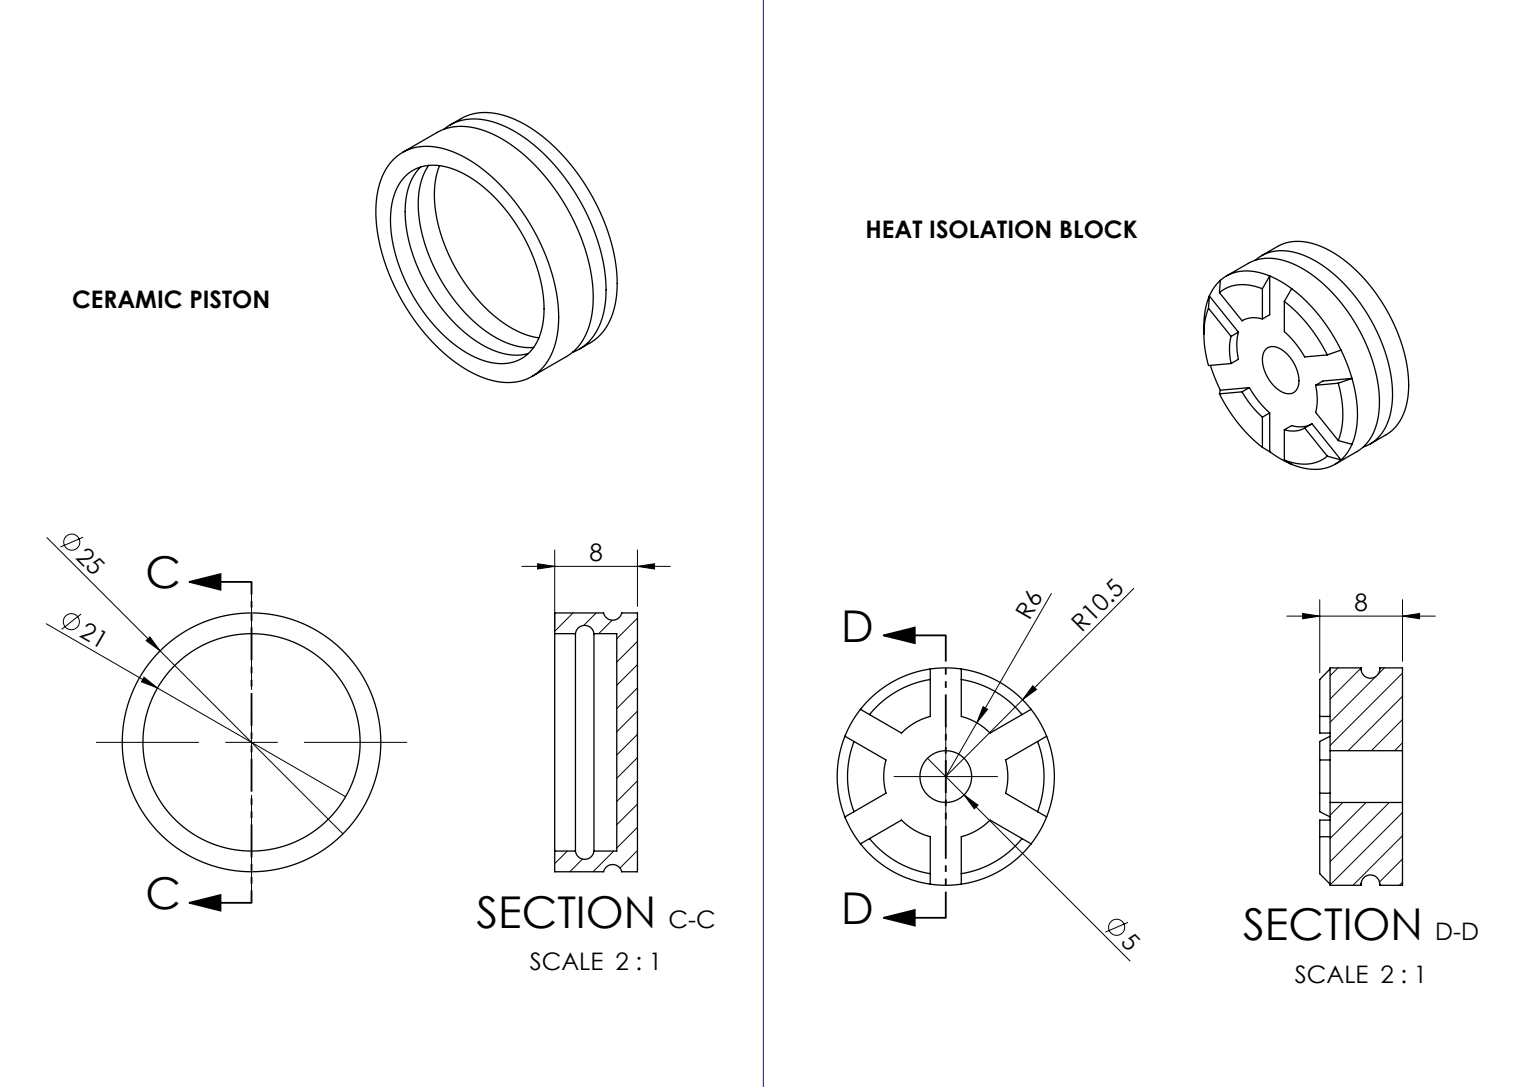
ISO-10303-21;
HEADER;
FILE_DESCRIPTION (('STEP AP214'),
    '1' );
FILE_NAME ('heat isolation block.step',
    '2026-09-24T10:28:59',
    ( '' ),
    ( '' ),
    'SwSTEP 2.0',
    'SolidWorks 2026',
    '' );
FILE_SCHEMA (( 'AUTOMOTIVE_DESIGN' ));
ENDSEC;

DATA;
#9=CARTESIAN_POINT ( 'NONE',  ( -4.281152949374567029, -4.203775615332181914, -2.000000000000000000 ) ) ;
#15=( GEOMETRIC_REPRESENTATION_CONTEXT ( 3 ) GLOBAL_UNCERTAINTY_ASSIGNED_CONTEXT ( ( #3731 ) ) GLOBAL_UNIT_ASSIGNED_CONTEXT ( ( #3713, #4977, #14697 ) ) REPRESENTATION_CONTEXT ( 'NONE', 'WORKASPACE' ) );
#20=CIRCLE ( 'NONE', #5504, 10.50000000000000000 ) ;
#39=CONICAL_SURFACE ( 'NONE', #2378, 9.500000000000001776, 0.7853981633974465026 ) ;
#43=VERTEX_POINT ( 'NONE', #14629 ) ;
#62=CIRCLE ( 'NONE', #4991, 10.50000000000000000 ) ;
#69=DIRECTION ( 'NONE',  ( 0.5000000000000038858, 0.8660254037844363761, 0.000000000000000000 ) ) ;
#71=DIRECTION ( 'NONE',  ( 1.000000000000000000, 0.000000000000000000, 0.000000000000000000 ) ) ;
#73=CARTESIAN_POINT ( 'NONE',  ( 0.000000000000000000, 0.000000000000000000, -2.000000000000000000 ) ) ;
#80=CIRCLE ( 'NONE', #3851, 6.000000000000000888 ) ;
#85=EDGE_LOOP ( 'NONE', ( #16844, #9736, #6237, #10207 ) ) ;
#89=ORIENTED_EDGE ( 'NONE', *, *, #2806, .T. ) ;
#104=CARTESIAN_POINT ( 'NONE',  ( 8.249999999999971578, -6.495190528383328221, -3.000000000000002665 ) ) ;
#107=DIRECTION ( 'NONE',  ( 0.000000000000000000, 0.000000000000000000, -1.000000000000000000 ) ) ;
#128=LINE ( 'NONE', #15357, #5139 ) ;
#130=DIRECTION ( 'NONE',  ( 0.8660254037844432595, 0.4999999999999921174, 0.000000000000000000 ) ) ;
#137=EDGE_CURVE ( 'NONE', #13969, #14024, #12150, .T. ) ;
#143=CARTESIAN_POINT ( 'NONE',  ( 0.000000000000000000, 0.000000000000000000, -3.000000000000000000 ) ) ;
#152=ORIENTED_EDGE ( 'NONE', *, *, #13921, .T. ) ;
#174=ORIENTED_EDGE ( 'NONE', *, *, #13419, .F. ) ;
#189=FACE_OUTER_BOUND ( 'NONE', #16988, .T. ) ;
#198=ORIENTED_EDGE ( 'NONE', *, *, #5351, .T. ) ;
#202=DIRECTION ( 'NONE',  ( -1.000000000000000000, 0.000000000000000000, 0.000000000000000000 ) ) ;
#207=EDGE_LOOP ( 'NONE', ( #11422, #8377, #17595, #13814 ) ) ;
#219=VECTOR ( 'NONE', #12447, 1000.000000000000000 ) ;
#251=CIRCLE ( 'NONE', #10368, 10.50000000000000000 ) ;
#318=ORIENTED_EDGE ( 'NONE', *, *, #17763, .T. ) ;
#357=AXIS2_PLACEMENT_3D ( 'NONE', #9695, #13538, #6726 ) ;
#359=CARTESIAN_POINT ( 'NONE',  ( 0.000000000000000000, 0.000000000000000000, -2.000000000000000000 ) ) ;
#360=AXIS2_PLACEMENT_3D ( 'NONE', #8254, #1099, #13788 ) ;
#369=DIRECTION ( 'NONE',  ( 0.000000000000000000, 0.000000000000000000, 1.000000000000000000 ) ) ;
#371=LINE ( 'NONE', #5878, #16268 ) ;
#388=ADVANCED_FACE ( 'NONE', ( #5520 ), #11038, .F. ) ;
#394=VECTOR ( 'NONE', #8237, 1000.000000000000114 ) ;
#409=CARTESIAN_POINT ( 'NONE',  ( -8.249999999999923617, 6.495190528383386841, -3.000000000000002665 ) ) ;
#415=CARTESIAN_POINT ( 'NONE',  ( -10.50000000000000000, -1.591841644184202181E-21, -6.005572809000082835 ) ) ;
#417=ORIENTED_EDGE ( 'NONE', *, *, #1398, .F. ) ;
#427=CARTESIAN_POINT ( 'NONE',  ( -8.874038404635992805, -3.391377654146690013, -2.000000000000000000 ) ) ;
#439=EDGE_LOOP ( 'NONE', ( #6272, #4236, #9102, #14227 ) ) ;
#467=CARTESIAN_POINT ( 'NONE',  ( -5.781152949374543937, -1.605699403978851247, -2.000000000000000000 ) ) ;
#470=PLANE ( 'NONE',  #13831 ) ;
#480=EDGE_CURVE ( 'NONE', #2781, #625, #723, .T. ) ;
#489=PLANE ( 'NONE',  #1672 ) ;
#504=DIRECTION ( 'NONE',  ( 1.000000000000000000, 0.000000000000000000, 0.000000000000000000 ) ) ;
#509=ORIENTED_EDGE ( 'NONE', *, *, #6536, .T. ) ;
#515=CARTESIAN_POINT ( 'NONE',  ( 1.500000000000000000, -10.39230484541326405, -3.000000000000000000 ) ) ;
#544=CARTESIAN_POINT ( 'NONE',  ( 0.000000000000000000, 0.000000000000000000, -10.00000000000000000 ) ) ;
#557=EDGE_CURVE ( 'NONE', #11479, #14024, #4933, .T. ) ;
#571=DIRECTION ( 'NONE',  ( 1.000000000000000000, 0.000000000000000000, -0.000000000000000000 ) ) ;
#578=EDGE_CURVE ( 'NONE', #729, #4780, #14420, .T. ) ;
#579=VERTEX_POINT ( 'NONE', #6435 ) ;
#601=CARTESIAN_POINT ( 'NONE',  ( 1.296864337298335788E-21, -1.182044466681725685E-21, -6.899999999999998579 ) ) ;
#606=DIRECTION ( 'NONE',  ( 0.4999999999999921174, -0.8660254037844432595, -0.000000000000000000 ) ) ;
#625=VERTEX_POINT ( 'NONE', #4973 ) ;
#634=CARTESIAN_POINT ( 'NONE',  ( 5.781152949374520844, -1.605699403978932294, -1.901951201008075243 ) ) ;
#643=ORIENTED_EDGE ( 'NONE', *, *, #10821, .T. ) ;
#667=VECTOR ( 'NONE', #5113, 1000.000000000000000 ) ;
#674=LINE ( 'NONE', #6104, #12815 ) ;
#676=DIRECTION ( 'NONE',  ( 1.000000000000000000, 0.000000000000000000, -0.000000000000000000 ) ) ;
#688=DIRECTION ( 'NONE',  ( 0.000000000000000000, 0.000000000000000000, 1.000000000000000000 ) ) ;
#700=CARTESIAN_POINT ( 'NONE',  ( 2.500000000000000000, 0.000000000000000000, -10.00000000000000000 ) ) ;
#710=EDGE_CURVE ( 'NONE', #12766, #3366, #5509, .T. ) ;
#723=LINE ( 'NONE', #1918, #13063 ) ;
#729=VERTEX_POINT ( 'NONE', #6905 ) ;
#744=FACE_OUTER_BOUND ( 'NONE', #10937, .T. ) ;
#749=LINE ( 'NONE', #17278, #4040 ) ;
#752=EDGE_CURVE ( 'NONE', #1869, #2438, #6375, .T. ) ;
#764=CARTESIAN_POINT ( 'NONE',  ( -4.281152949374478212, 4.203775615332272508, -3.000000000000000888 ) ) ;
#819=CARTESIAN_POINT ( 'NONE',  ( -7.958171371210956302, 6.326703190994831694, -2.666481567098320404 ) ) ;
#821=EDGE_LOOP ( 'NONE', ( #12913, #198, #11384, #8365 ) ) ;
#842=AXIS2_PLACEMENT_3D ( 'NONE', #9935, #3246, #7424 ) ;
#848=CIRCLE ( 'NONE', #14764, 9.500000000000001776 ) ;
#849=FACE_OUTER_BOUND ( 'NONE', #85, .T. ) ;
#851=CARTESIAN_POINT ( 'NONE',  ( 0.000000000000000000, 0.000000000000000000, -3.000000000000002665 ) ) ;
#912=ORIENTED_EDGE ( 'NONE', *, *, #15355, .F. ) ;
#915=ADVANCED_FACE ( 'NONE', ( #1453 ), #39, .T. ) ;
#932=FACE_OUTER_BOUND ( 'NONE', #17119, .T. ) ;
#937=CIRCLE ( 'NONE', #357, 6.000000000000000888 ) ;
#940=VECTOR ( 'NONE', #5062, 1000.000000000000000 ) ;
#946=CARTESIAN_POINT ( 'NONE',  ( 1.500000000000000000, -11.00000000000000000, -9.708203932499369415 ) ) ;
#1001=DIRECTION ( 'NONE',  ( 0.000000000000000000, 0.000000000000000000, -1.000000000000000000 ) ) ;
#1049=ORIENTED_EDGE ( 'NONE', *, *, #11408, .F. ) ;
#1060=CARTESIAN_POINT ( 'NONE',  ( -10.50000000000000000, 0.000000000000000000, -2.000000000000000000 ) ) ;
#1069=VERTEX_POINT ( 'NONE', #8885 ) ;
#1099=DIRECTION ( 'NONE',  ( -0.000000000000000000, -0.000000000000000000, 1.000000000000000000 ) ) ;
#1136=AXIS2_PLACEMENT_3D ( 'NONE', #7243, #8688, #3068 ) ;
#1187=EDGE_LOOP ( 'NONE', ( #16383, #1379, #6856, #3698 ) ) ;
#1190=LINE ( 'NONE', #7567, #15018 ) ;
#1192=AXIS2_PLACEMENT_3D ( 'NONE', #16349, #13436, #5076 ) ;
#1198=VERTEX_POINT ( 'NONE', #8051 ) ;
#1209=AXIS2_PLACEMENT_3D ( 'NONE', #2238, #17500, #17400 ) ;
#1235=CIRCLE ( 'NONE', #11336, 2.500000000000000000 ) ;
#1240=ADVANCED_FACE ( 'NONE', ( #2709 ), #17880, .T. ) ;
#1258=DIRECTION ( 'NONE',  ( -0.8660254037844397068, -0.4999999999999981126, 0.000000000000000000 ) ) ;
#1288=EDGE_LOOP ( 'NONE', ( #15134, #15555, #15815, #8257 ) ) ;
#1290=CARTESIAN_POINT ( 'NONE',  ( -1.500000000000000000, -10.39230484541326405, -3.000000000000002665 ) ) ;
#1307=DIRECTION ( 'NONE',  ( 0.8660254037844397068, 0.4999999999999981126, -0.000000000000000000 ) ) ;
#1308=CARTESIAN_POINT ( 'NONE',  ( 0.000000000000000000, 0.000000000000000000, -2.000000000000000000 ) ) ;
#1332=ORIENTED_EDGE ( 'NONE', *, *, #12922, .F. ) ;
#1344=FACE_OUTER_BOUND ( 'NONE', #5620, .T. ) ;
#1350=ORIENTED_EDGE ( 'NONE', *, *, #12982, .T. ) ;
#1360=CARTESIAN_POINT ( 'NONE',  ( 9.750000000000010658, 3.897114317029950037, -3.000000000000002665 ) ) ;
#1368=AXIS2_PLACEMENT_3D ( 'NONE', #5699, #11216, #16788 ) ;
#1372=CARTESIAN_POINT ( 'NONE',  ( 7.958171371211001599, -6.326703190994774850, -2.666481567098319960 ) ) ;
#1379=ORIENTED_EDGE ( 'NONE', *, *, #5330, .F. ) ;
#1392=DIRECTION ( 'NONE',  ( 1.000000000000000000, 0.000000000000000000, 0.000000000000000000 ) ) ;
#1398=EDGE_CURVE ( 'NONE', #9792, #11171, #4666, .T. ) ;
#1408=PRODUCT_DEFINITION_CONTEXT ( 'detailed design', #12580, 'design' ) ;
#1414=CARTESIAN_POINT ( 'NONE',  ( 10.37836969302994028, -0.6704047395399680420, -6.899999999999998579 ) ) ;
#1421=VERTEX_POINT ( 'NONE', #13936 ) ;
#1431=AXIS2_PLACEMENT_3D ( 'NONE', #10215, #17040, #3248 ) ;
#1453=FACE_OUTER_BOUND ( 'NONE', #15787, .T. ) ;
#1455=CARTESIAN_POINT ( 'NONE',  ( -1.500000000000000000, 10.39230484541326227, -3.000000000000000000 ) ) ;
#1470=AXIS2_PLACEMENT_3D ( 'NONE', #15599, #1647, #12691 ) ;
#1472=CARTESIAN_POINT ( 'NONE',  ( -1.499999999999999778, 9.380831519646861238, -2.000000000000000000 ) ) ;
#1512=EDGE_CURVE ( 'NONE', #11483, #15072, #14540, .T. ) ;
#1523=CARTESIAN_POINT ( 'NONE',  ( 1.499999999999999778, -9.718191103688257115, -2.333127728361105380 ) ) ;
#1526=ORIENTED_EDGE ( 'NONE', *, *, #7540, .T. ) ;
#1553=DIRECTION ( 'NONE',  ( 0.000000000000000000, 0.000000000000000000, -1.000000000000000000 ) ) ;
#1566=ORIENTED_EDGE ( 'NONE', *, *, #10647, .T. ) ;
#1572=VERTEX_POINT ( 'NONE', #5185 ) ;
#1580=CARTESIAN_POINT ( 'NONE',  ( 5.781152949374531502, 1.605699403978890771, -1.901951201008075243 ) ) ;
#1600=ADVANCED_FACE ( 'NONE', ( #9886 ), #12895, .F. ) ;
#1615=VERTEX_POINT ( 'NONE', #8632 ) ;
#1626=DIRECTION ( 'NONE',  ( 0.000000000000000000, 0.000000000000000000, -1.000000000000000000 ) ) ;
#1647=DIRECTION ( 'NONE',  ( 0.4999999999999921174, -0.8660254037844432595, -0.000000000000000000 ) ) ;
#1655=CARTESIAN_POINT ( 'NONE',  ( -1.500000000000000000, 10.05532945112458698, -2.666480854966546854 ) ) ;
#1668=ADVANCED_FACE ( 'NONE', ( #744 ), #12214, .F. ) ;
#1672=AXIS2_PLACEMENT_3D ( 'NONE', #7393, #12994, #6000 ) ;
#1699=CARTESIAN_POINT ( 'NONE',  ( 1.499999999999999778, -9.380831519646861238, -2.000000000000000000 ) ) ;
#1700=EDGE_CURVE ( 'NONE', #17480, #7830, #17463, .T. ) ;
#1727=FACE_OUTER_BOUND ( 'NONE', #3816, .T. ) ;
#1738=CARTESIAN_POINT ( 'NONE',  ( -8.776279441628744848, 6.799038105676760146, -11.72793873352925331 ) ) ;
#1745=CARTESIAN_POINT ( 'NONE',  ( 1.500000000000000666, 5.809475019311125976, -3.000000000000000000 ) ) ;
#1757=PLANE ( 'NONE',  #3505 ) ;
#1768=CARTESIAN_POINT ( 'NONE',  ( 0.000000000000000000, 0.000000000000000000, -2.000000000000000000 ) ) ;
#1772=DIRECTION ( 'NONE',  ( 1.224646799147353207E-16, -1.000000000000000000, 0.000000000000000000 ) ) ;
#1786=DIRECTION ( 'NONE',  ( -0.8660254037844397068, -0.4999999999999981126, 0.000000000000000000 ) ) ;
#1798=CARTESIAN_POINT ( 'NONE',  ( -10.37836969302994028, 0.6704047395399693743, -6.899999999999998579 ) ) ;
#1802=AXIS2_PLACEMENT_3D ( 'NONE', #10064, #17179, #202 ) ;
#1809=PLANE ( 'NONE',  #1136 ) ;
#1842=VECTOR ( 'NONE', #5538, 1000.000000000000000 ) ;
#1843=AXIS2_PLACEMENT_3D ( 'NONE', #12222, #9657, #2789 ) ;
#1849=CIRCLE ( 'NONE', #1431, 10.50000000000000000 ) ;
#1851=EDGE_LOOP ( 'NONE', ( #4202, #12524, #6400, #11426 ) ) ;
#1862=CIRCLE ( 'NONE', #6762, 9.500000000000000000 ) ;
#1867=ORIENTED_EDGE ( 'NONE', *, *, #13233, .T. ) ;
#1869=VERTEX_POINT ( 'NONE', #1455 ) ;
#1875=CIRCLE ( 'NONE', #3312, 2.500000000000000000 ) ;
#1918=CARTESIAN_POINT ( 'NONE',  ( 8.776279441628840772, 6.799038105676637578, -3.000000000000000888 ) ) ;
#1929=DIRECTION ( 'NONE',  ( -0.000000000000000000, -0.000000000000000000, -1.000000000000000000 ) ) ;
#1936=ADVANCED_FACE ( 'NONE', ( #10861 ), #2733, .F. ) ;
#1938=ORIENTED_EDGE ( 'NONE', *, *, #9820, .F. ) ;
#1984=CARTESIAN_POINT ( 'NONE',  ( 0.000000000000000000, 0.000000000000000000, -2.000000000000000000 ) ) ;
#1993=ORIENTED_EDGE ( 'NONE', *, *, #14425, .F. ) ;
#1996=EDGE_CURVE ( 'NONE', #14070, #1615, #10473, .T. ) ;
#2030=DIRECTION ( 'NONE',  ( -1.000000000000000000, 0.000000000000000000, 0.000000000000000000 ) ) ;
#2038=CYLINDRICAL_SURFACE ( 'NONE', #14415, 10.50000000000000000 ) ;
#2040=DIRECTION ( 'NONE',  ( 1.000000000000000000, 0.000000000000000000, 0.000000000000000000 ) ) ;
#2042=DIRECTION ( 'NONE',  ( 0.000000000000000000, 0.000000000000000000, -1.000000000000000000 ) ) ;
#2053=DIRECTION ( 'NONE',  ( 1.000000000000000000, 0.000000000000000000, 0.000000000000000000 ) ) ;
#2071=LINE ( 'NONE', #700, #12556 ) ;
#2076=ADVANCED_FACE ( 'NONE', ( #5791 ), #16001, .T. ) ;
#2083=DIRECTION ( 'NONE',  ( -1.000000000000000000, 0.000000000000000000, 0.000000000000000000 ) ) ;
#2099=CIRCLE ( 'NONE', #13645, 10.50000000000000000 ) ;
#2109=EDGE_CURVE ( 'NONE', #3845, #13908, #12877, .T. ) ;
#2116=EDGE_LOOP ( 'NONE', ( #14184, #10060, #9084, #13984 ) ) ;
#2125=CIRCLE ( 'NONE', #4141, 10.50000000000000000 ) ;
#2129=VECTOR ( 'NONE', #4034, 999.9999999999998863 ) ;
#2141=CARTESIAN_POINT ( 'NONE',  ( 0.000000000000000000, 0.000000000000000000, -3.000000000000002665 ) ) ;
#2172=CYLINDRICAL_SURFACE ( 'NONE', #7782, 6.000000000000000888 ) ;
#2184=DIRECTION ( 'NONE',  ( -0.000000000000000000, -0.000000000000000000, -1.000000000000000000 ) ) ;
#2196=EDGE_LOOP ( 'NONE', ( #15610, #7635, #5937, #16842 ) ) ;
#2220=EDGE_CURVE ( 'NONE', #15040, #7588, #15871, .T. ) ;
#2226=VERTEX_POINT ( 'NONE', #13147 ) ;
#2231=EDGE_CURVE ( 'NONE', #15452, #4832, #62, .T. ) ;
#2238=CARTESIAN_POINT ( 'NONE',  ( 8.472608240843633681E-22, -7.722472891792491889E-22, -7.794427190999915211 ) ) ;
#2248=CARTESIAN_POINT ( 'NONE',  ( 0.000000000000000000, 0.000000000000000000, -3.000000000000002665 ) ) ;
#2250=CARTESIAN_POINT ( 'NONE',  ( 10.27627944162880702, -4.200961894323389956, -11.72793873352923910 ) ) ;
#2280=FILL_AREA_STYLE ('',( #9238 ) ) ;
#2308=ADVANCED_FACE ( 'NONE', ( #1344 ), #13506, .T. ) ;
#2309=CIRCLE ( 'NONE', #4601, 10.50000000000000000 ) ;
#2319=DIRECTION ( 'NONE',  ( 1.000000000000000000, 4.440892098500626951E-15, 0.000000000000000000 ) ) ;
#2322=AXIS2_PLACEMENT_3D ( 'NONE', #6054, #3437, #5876 ) ;
#2343=DIRECTION ( 'NONE',  ( 0.5000000000000038858, 0.8660254037844363761, 0.000000000000000000 ) ) ;
#2346=DIRECTION ( 'NONE',  ( -1.000000000000000000, 0.000000000000000000, 0.000000000000000000 ) ) ;
#2371=CARTESIAN_POINT ( 'NONE',  ( 0.000000000000000000, 0.000000000000000000, -3.000000000000002665 ) ) ;
#2374=SURFACE_STYLE_USAGE ( .BOTH. , #14785 ) ;
#2378=AXIS2_PLACEMENT_3D ( 'NONE', #12332, #17897, #10945 ) ;
#2389=AXIS2_PLACEMENT_3D ( 'NONE', #16083, #3561, #10523 ) ;
#2421=ORIENTED_EDGE ( 'NONE', *, *, #3769, .F. ) ;
#2438=VERTEX_POINT ( 'NONE', #16490 ) ;
#2454=( NAMED_UNIT ( * ) PLANE_ANGLE_UNIT ( ) SI_UNIT ( $, .RADIAN. ) );
#2462=EDGE_CURVE ( 'NONE', #14411, #17313, #11338, .T. ) ;
#2529=LINE ( 'NONE', #15127, #394 ) ;
#2540=ORIENTED_EDGE ( 'NONE', *, *, #5351, .F. ) ;
#2546=CARTESIAN_POINT ( 'NONE',  ( 8.776279441628796363, -6.799038105676699750, -3.000000000000000888 ) ) ;
#2558=DIRECTION ( 'NONE',  ( 1.000000000000000000, 7.105427357601001859E-15, 0.000000000000000000 ) ) ;
#2566=AXIS2_PLACEMENT_3D ( 'NONE', #17401, #3402, #11731 ) ;
#2637=CARTESIAN_POINT ( 'NONE',  ( 8.874038404635971489, 3.391377654146752629, -2.000000000000000000 ) ) ;
#2645=EDGE_CURVE ( 'NONE', #9826, #1069, #3570, .T. ) ;
#2653=AXIS2_PLACEMENT_3D ( 'NONE', #11618, #6546, #17738 ) ;
#2669=AXIS2_PLACEMENT_3D ( 'NONE', #11406, #1553, #12604 ) ;
#2709=FACE_OUTER_BOUND ( 'NONE', #4089, .T. ) ;
#2715=SHAPE_REPRESENTATION_RELATIONSHIP ( 'NONE' , 'NONE' ,  #12598, #7018 ) ;
#2733=CYLINDRICAL_SURFACE ( 'NONE', #360, 2.500000000000000000 ) ;
#2740=CARTESIAN_POINT ( 'NONE',  ( 4.281152949374537720, 4.203775615332211224, -3.000000000000000888 ) ) ;
#2780=ORIENTED_EDGE ( 'NONE', *, *, #13626, .F. ) ;
#2781=VERTEX_POINT ( 'NONE', #2740 ) ;
#2789=DIRECTION ( 'NONE',  ( -0.9979201627913402151, 0.06446199418653550395, 5.311609029246448998E-22 ) ) ;
#2798=CARTESIAN_POINT ( 'NONE',  ( -1.500000000000000222, -9.718191103688257115, -2.333127728361105824 ) ) ;
#2806=EDGE_CURVE ( 'NONE', #13908, #625, #6456, .T. ) ;
#2839=VERTEX_POINT ( 'NONE', #3278 ) ;
#2852=VECTOR ( 'NONE', #15204, 1000.000000000000000 ) ;
#2868=CARTESIAN_POINT ( 'NONE',  ( 8.776279441628840772, 6.799038105676637578, -11.72793873352922489 ) ) ;
#2873=DIRECTION ( 'NONE',  ( -0.8660254037844363761, 0.5000000000000038858, 0.000000000000000000 ) ) ;
#2910=ORIENTED_EDGE ( 'NONE', *, *, #10359, .T. ) ;
#2921=CARTESIAN_POINT ( 'NONE',  ( -9.480241546517731877, 0.6123889447720874957, -6.899999999999998579 ) ) ;
#2957=AXIS2_PLACEMENT_3D ( 'NONE', #1798, #10206, #9832 ) ;
#2969=ORIENTED_EDGE ( 'NONE', *, *, #10235, .T. ) ;
#2987=DIRECTION ( 'NONE',  ( 1.000000000000000000, 0.000000000000000000, 0.000000000000000000 ) ) ;
#2988=ADVANCED_FACE ( 'NONE', ( #8616 ), #14148, .T. ) ;
#3008=CARTESIAN_POINT ( 'NONE',  ( 7.666200962222293747, -6.158133996769738161, -2.333128398347827481 ) ) ;
#3062=DIRECTION ( 'NONE',  ( -0.000000000000000000, -0.000000000000000000, -1.000000000000000000 ) ) ;
#3068=DIRECTION ( 'NONE',  ( -0.8660254037844397068, -0.4999999999999981126, 0.000000000000000000 ) ) ;
#3101=DIRECTION ( 'NONE',  ( 0.000000000000000000, 0.000000000000000000, 1.000000000000000000 ) ) ;
#3104=AXIS2_PLACEMENT_3D ( 'NONE', #11983, #16358, #17566 ) ;
#3160=ORIENTED_EDGE ( 'NONE', *, *, #10235, .F. ) ;
#3205=AXIS2_PLACEMENT_3D ( 'NONE', #10231, #10312, #10043 ) ;
#3220=SHAPE_DEFINITION_REPRESENTATION ( #17387, #12598 ) ;
#3229=VECTOR ( 'NONE', #17641, 999.9999999999998863 ) ;
#3246=DIRECTION ( 'NONE',  ( 0.000000000000000000, 0.000000000000000000, -1.000000000000000000 ) ) ;
#3248=DIRECTION ( 'NONE',  ( 1.000000000000000000, 0.000000000000000000, 0.000000000000000000 ) ) ;
#3278=CARTESIAN_POINT ( 'NONE',  ( -4.281152949374479100, 4.203775615332271620, -2.000000000000000000 ) ) ;
#3292=EDGE_CURVE ( 'NONE', #11171, #14411, #8219, .T. ) ;
#3306=DIRECTION ( 'NONE',  ( 0.000000000000000000, 0.000000000000000000, -1.000000000000000000 ) ) ;
#3309=DIRECTION ( 'NONE',  ( -0.000000000000000000, -0.000000000000000000, -1.000000000000000000 ) ) ;
#3312=AXIS2_PLACEMENT_3D ( 'NONE', #5444, #12434, #16617 ) ;
#3319=CARTESIAN_POINT ( 'NONE',  ( -7.958171371211089529, -6.326703190994665604, -2.666481567098319516 ) ) ;
#3331=DIRECTION ( 'NONE',  ( -0.000000000000000000, -0.000000000000000000, 1.000000000000000000 ) ) ;
#3344=ORIENTED_EDGE ( 'NONE', *, *, #5310, .T. ) ;
#3357=EDGE_CURVE ( 'NONE', #1615, #14070, #251, .T. ) ;
#3362=FACE_OUTER_BOUND ( 'NONE', #5487, .T. ) ;
#3366=VERTEX_POINT ( 'NONE', #427 ) ;
#3367=ADVANCED_FACE ( 'NONE', ( #11823 ), #11513, .F. ) ;
#3388=CARTESIAN_POINT ( 'NONE',  ( 10.50000000000000000, 1.285879139104720831E-15, -2.000000000000000000 ) ) ;
#3395=LINE ( 'NONE', #7572, #1842 ) ;
#3402=DIRECTION ( 'NONE',  ( -5.026720092345836698E-22, 4.581671729415424240E-22, -1.000000000000000000 ) ) ;
#3404=VECTOR ( 'NONE', #7432, 1000.000000000000000 ) ;
#3405=ORIENTED_EDGE ( 'NONE', *, *, #10870, .F. ) ;
#3422=FACE_OUTER_BOUND ( 'NONE', #8222, .T. ) ;
#3437=DIRECTION ( 'NONE',  ( 0.000000000000000000, 0.000000000000000000, -1.000000000000000000 ) ) ;
#3471=CARTESIAN_POINT ( 'NONE',  ( -2.500000000000000000, 3.061616997868383141E-16, -10.00000000000000000 ) ) ;
#3505=AXIS2_PLACEMENT_3D ( 'NONE', #14357, #12986, #571 ) ;
#3506=DIRECTION ( 'NONE',  ( 1.000000000000000000, 0.000000000000000000, 0.000000000000000000 ) ) ;
#3525=ORIENTED_EDGE ( 'NONE', *, *, #17843, .F. ) ;
#3540=AXIS2_PLACEMENT_3D ( 'NONE', #544, #16784, #14056 ) ;
#3554=AXIS2_PLACEMENT_3D ( 'NONE', #6267, #14796, #11882 ) ;
#3561=DIRECTION ( 'NONE',  ( -5.026720092345836698E-22, 4.581671729415424240E-22, -1.000000000000000000 ) ) ;
#3570=LINE ( 'NONE', #3471, #8184 ) ;
#3575=AXIS2_PLACEMENT_3D ( 'NONE', #5095, #17575, #9272 ) ;
#3577=ORIENTED_EDGE ( 'NONE', *, *, #11050, .T. ) ;
#3589=DIRECTION ( 'NONE',  ( 1.000000000000000000, 0.000000000000000000, 0.000000000000000000 ) ) ;
#3600=DIRECTION ( 'NONE',  ( -1.000000000000000000, 0.000000000000000000, 0.000000000000000000 ) ) ;
#3609=PLANE ( 'NONE',  #13979 ) ;
#3615=PRODUCT ( 'heat isolation block', 'heat isolation block', '', ( #13914 ) ) ;
#3643=EDGE_LOOP ( 'NONE', ( #3916, #14619, #4515, #16461, #2780 ) ) ;
#3665=CARTESIAN_POINT ( 'NONE',  ( -9.458171371211065548, -3.728626979641334493, -2.666481567098320404 ) ) ;
#3684=CARTESIAN_POINT ( 'NONE',  ( 1.500000000000000000, 10.05532945112459053, -2.666480854966549519 ) ) ;
#3697=ORIENTED_EDGE ( 'NONE', *, *, #578, .F. ) ;
#3698=ORIENTED_EDGE ( 'NONE', *, *, #14726, .F. ) ;
#3713=( LENGTH_UNIT ( ) NAMED_UNIT ( * ) SI_UNIT ( .MILLI., .METRE. ) );
#3715=CIRCLE ( 'NONE', #6012, 0.9000000000000003553 ) ;
#3731=UNCERTAINTY_MEASURE_WITH_UNIT (LENGTH_MEASURE( 1.000000000000000082E-05 ), #3713, 'distance_accuracy_value', 'NONE');
#3752=CARTESIAN_POINT ( 'NONE',  ( -1.500000000000000000, -11.00000000000000000, -2.000000000000000000 ) ) ;
#3758=CARTESIAN_POINT ( 'NONE',  ( 7.374038404635976818, 5.989453865500072638, -2.000000000000000000 ) ) ;
#3759=B_SPLINE_CURVE_WITH_KNOTS ( 'NONE', 3,
 ( #17890, #13856, #2798, #10934 ),
 .UNSPECIFIED., .F., .F.,
 ( 4, 4 ),
 ( 0.007932485430080135971, 0.009354825709699443950 ),
 .UNSPECIFIED. ) ;
#3769=EDGE_CURVE ( 'NONE', #15072, #12450, #6094, .T. ) ;
#3773=VERTEX_POINT ( 'NONE', #5910 ) ;
#3775=CARTESIAN_POINT ( 'NONE',  ( 1.500000000000000000, 10.39230484541326227, -3.000000000000000000 ) ) ;
#3785=CARTESIAN_POINT ( 'NONE',  ( 10.50000000000000000, 1.285879139104720831E-15, -3.000000000000002665 ) ) ;
#3802=ADVANCED_FACE ( 'NONE', ( #15624 ), #14272, .T. ) ;
#3811=VECTOR ( 'NONE', #15051, 999.9999999999998863 ) ;
#3816=EDGE_LOOP ( 'NONE', ( #4598, #10832, #4008, #10200 ) ) ;
#3819=ORIENTED_EDGE ( 'NONE', *, *, #4860, .T. ) ;
#3830=AXIS2_PLACEMENT_3D ( 'NONE', #6269, #7906, #11885 ) ;
#3845=VERTEX_POINT ( 'NONE', #1745 ) ;
#3848=VECTOR ( 'NONE', #1772, 1000.000000000000000 ) ;
#3851=AXIS2_PLACEMENT_3D ( 'NONE', #17013, #7216, #8477 ) ;
#3857=AXIS2_PLACEMENT_3D ( 'NONE', #11830, #606, #13117 ) ;
#3887=DIRECTION ( 'NONE',  ( 0.000000000000000000, 0.000000000000000000, 1.000000000000000000 ) ) ;
#3916=ORIENTED_EDGE ( 'NONE', *, *, #4860, .F. ) ;
#3957=CARTESIAN_POINT ( 'NONE',  ( 1.500000000000000222, 9.380831519646861238, -2.000000000000000000 ) ) ;
#3964=ORIENTED_EDGE ( 'NONE', *, *, #16776, .T. ) ;
#3971=VECTOR ( 'NONE', #16088, 1000.000000000000000 ) ;
#3986=CIRCLE ( 'NONE', #10905, 10.50000000000000000 ) ;
#4008=ORIENTED_EDGE ( 'NONE', *, *, #12945, .F. ) ;
#4017=ORIENTED_EDGE ( 'NONE', *, *, #15259, .F. ) ;
#4020=CARTESIAN_POINT ( 'NONE',  ( -10.50000000000000000, 0.000000000000000000, -10.00000000000000000 ) ) ;
#4034=DIRECTION ( 'NONE',  ( -0.7071067811865462405, 0.000000000000000000, -0.7071067811865489050 ) ) ;
#4040=VECTOR ( 'NONE', #15896, 1000.000000000000114 ) ;
#4047=AXIS2_PLACEMENT_3D ( 'NONE', #5466, #15185, #6927 ) ;
#4048=ORIENTED_EDGE ( 'NONE', *, *, #15785, .T. ) ;
#4056=DIRECTION ( 'NONE',  ( 1.000000000000000000, 0.000000000000000000, 0.000000000000000000 ) ) ;
#4069=EDGE_CURVE ( 'NONE', #15072, #2226, #11486, .T. ) ;
#4078=LINE ( 'NONE', #2546, #3229 ) ;
#4089=EDGE_LOOP ( 'NONE', ( #7110, #11157, #11633, #17145, #10471, #8655 ) ) ;
#4099=EDGE_CURVE ( 'NONE', #1198, #579, #8316, .T. ) ;
#4107=EDGE_CURVE ( 'NONE', #1572, #17008, #13634, .T. ) ;
#4131=CARTESIAN_POINT ( 'NONE',  ( 0.000000000000000000, 0.000000000000000000, -1.901951201008075243 ) ) ;
#4141=AXIS2_PLACEMENT_3D ( 'NONE', #2141, #2042, #11634 ) ;
#4147=EDGE_CURVE ( 'NONE', #11147, #14109, #3986, .T. ) ;
#4191=EDGE_CURVE ( 'NONE', #14530, #1198, #7387, .T. ) ;
#4202=ORIENTED_EDGE ( 'NONE', *, *, #7943, .T. ) ;
#4236=ORIENTED_EDGE ( 'NONE', *, *, #15879, .T. ) ;
#4252=FACE_OUTER_BOUND ( 'NONE', #12699, .T. ) ;
#4255=ORIENTED_EDGE ( 'NONE', *, *, #9354, .F. ) ;
#4295=VECTOR ( 'NONE', #9727, 1000.000000000000000 ) ;
#4335=CIRCLE ( 'NONE', #8972, 6.000000000000000888 ) ;
#4379=CIRCLE ( 'NONE', #16830, 10.50000000000000000 ) ;
#4433=EDGE_LOOP ( 'NONE', ( #12591, #16245 ) ) ;
#4468=ORIENTED_EDGE ( 'NONE', *, *, #10158, .T. ) ;
#4484=EDGE_CURVE ( 'NONE', #13130, #1572, #5053, .T. ) ;
#4499=FACE_OUTER_BOUND ( 'NONE', #12923, .T. ) ;
#4515=ORIENTED_EDGE ( 'NONE', *, *, #1512, .F. ) ;
#4534=CARTESIAN_POINT ( 'NONE',  ( 0.000000000000000000, 0.000000000000000000, -2.000000000000000000 ) ) ;
#4544=ORIENTED_EDGE ( 'NONE', *, *, #13626, .T. ) ;
#4555=CONICAL_SURFACE ( 'NONE', #1368, 9.500000000000001776, 0.7853981633974465026 ) ;
#4557=CARTESIAN_POINT ( 'NONE',  ( 8.472608240843633681E-22, -7.722472891792491889E-22, -7.794427190999915211 ) ) ;
#4593=VERTEX_POINT ( 'NONE', #9713 ) ;
#4598=ORIENTED_EDGE ( 'NONE', *, *, #6536, .F. ) ;
#4601=AXIS2_PLACEMENT_3D ( 'NONE', #2371, #13507, #7889 ) ;
#4625=LINE ( 'NONE', #16793, #6902 ) ;
#4639=EDGE_CURVE ( 'NONE', #9144, #579, #128, .T. ) ;
#4654=ORIENTED_EDGE ( 'NONE', *, *, #752, .T. ) ;
#4655=CARTESIAN_POINT ( 'NONE',  ( 1.500000000000000000, -11.00000000000000000, -3.000000000000000000 ) ) ;
#4657=CARTESIAN_POINT ( 'NONE',  ( 0.000000000000000000, 0.000000000000000000, -1.901951201008075243 ) ) ;
#4666=CIRCLE ( 'NONE', #14810, 6.000000000000000888 ) ;
#4701=DIRECTION ( 'NONE',  ( -1.000000000000000000, 0.000000000000000000, 0.000000000000000000 ) ) ;
#4734=ADVANCED_FACE ( 'NONE', ( #14367 ), #489, .T. ) ;
#4735=DIRECTION ( 'NONE',  ( -0.000000000000000000, -0.000000000000000000, -1.000000000000000000 ) ) ;
#4738=ADVANCED_FACE ( 'NONE', ( #17098 ), #2038, .T. ) ;
#4739=ORIENTED_EDGE ( 'NONE', *, *, #15462, .F. ) ;
#4749=CARTESIAN_POINT ( 'NONE',  ( 0.000000000000000000, 0.000000000000000000, -2.000000000000000000 ) ) ;
#4750=CARTESIAN_POINT ( 'NONE',  ( -6.000000000000000888, 0.000000000000000000, -3.000000000000000000 ) ) ;
#4765=CARTESIAN_POINT ( 'NONE',  ( 1.500000000000000222, 9.380831519646861238, -2.000000000000000000 ) ) ;
#4780=VERTEX_POINT ( 'NONE', #10177 ) ;
#4788=EDGE_CURVE ( 'NONE', #12819, #43, #8619, .T. ) ;
#4814=CARTESIAN_POINT ( 'NONE',  ( -4.281152949374566141, -4.203775615332181026, -3.000000000000000888 ) ) ;
#4827=FACE_OUTER_BOUND ( 'NONE', #4433, .T. ) ;
#4832=VERTEX_POINT ( 'NONE', #409 ) ;
#4859=LINE ( 'NONE', #1060, #11852 ) ;
#4860=EDGE_CURVE ( 'NONE', #2226, #8959, #8646, .T. ) ;
#4883=FACE_OUTER_BOUND ( 'NONE', #8544, .T. ) ;
#4904=B_SPLINE_CURVE_WITH_KNOTS ( 'NONE', 3,
 ( #11646, #3319, #8932, #14474 ),
 .UNSPECIFIED., .F., .F.,
 ( 4, 4 ),
 ( 2.843119637691541009E-07, 0.001422633878257847061 ),
 .UNSPECIFIED. ) ;
#4915=ORIENTED_EDGE ( 'NONE', *, *, #5443, .F. ) ;
#4918=CARTESIAN_POINT ( 'NONE',  ( 0.000000000000000000, 0.000000000000000000, -2.000000000000000000 ) ) ;
#4933=CIRCLE ( 'NONE', #3205, 6.000000000000000888 ) ;
#4946=DIRECTION ( 'NONE',  ( -1.000000000000000000, 0.000000000000000000, 0.000000000000000000 ) ) ;
#4955=CARTESIAN_POINT ( 'NONE',  ( -7.374038404636016786, -5.989453865500021124, -2.000000000000000000 ) ) ;
#4961=ORIENTED_EDGE ( 'NONE', *, *, #3357, .T. ) ;
#4973=CARTESIAN_POINT ( 'NONE',  ( 8.250000000000014211, 6.495190528383269601, -3.000000000000000000 ) ) ;
#4977=( NAMED_UNIT ( * ) PLANE_ANGLE_UNIT ( ) SI_UNIT ( $, .RADIAN. ) );
#4980=VECTOR ( 'NONE', #6063, 1000.000000000000000 ) ;
#4991=AXIS2_PLACEMENT_3D ( 'NONE', #10582, #1001, #14613 ) ;
#5053=LINE ( 'NONE', #11676, #3404 ) ;
#5062=DIRECTION ( 'NONE',  ( 1.224646799147353207E-16, -1.000000000000000000, 0.000000000000000000 ) ) ;
#5076=DIRECTION ( 'NONE',  ( -1.000000000000000000, 0.000000000000000000, 0.000000000000000000 ) ) ;
#5092=CARTESIAN_POINT ( 'NONE',  ( 9.166200962222307069, -3.560057785416429255, -2.333128398347826593 ) ) ;
#5095=CARTESIAN_POINT ( 'NONE',  ( 0.000000000000000000, 0.000000000000000000, 0.000000000000000000 ) ) ;
#5096=DIRECTION ( 'NONE',  ( -1.224646799147353207E-16, 1.000000000000000000, 0.000000000000000000 ) ) ;
#5099=EDGE_CURVE ( 'NONE', #5285, #7960, #17353, .T. ) ;
#5104=ORIENTED_EDGE ( 'NONE', *, *, #12475, .T. ) ;
#5113=DIRECTION ( 'NONE',  ( 0.000000000000000000, 0.000000000000000000, -1.000000000000000000 ) ) ;
#5123=CARTESIAN_POINT ( 'NONE',  ( -5.781152949374542160, -1.605699403978850803, -3.000000000000000888 ) ) ;
#5134=ORIENTED_EDGE ( 'NONE', *, *, #16914, .T. ) ;
#5139=VECTOR ( 'NONE', #5641, 1000.000000000000000 ) ;
#5145=CARTESIAN_POINT ( 'NONE',  ( 0.000000000000000000, 0.000000000000000000, -2.000000000000000000 ) ) ;
#5155=DIRECTION ( 'NONE',  ( 1.000000000000000000, -1.776356839400250780E-14, 0.000000000000000000 ) ) ;
#5185=CARTESIAN_POINT ( 'NONE',  ( 5.781152949374531502, 1.605699403978890993, -2.000000000000000000 ) ) ;
#5195=ORIENTED_EDGE ( 'NONE', *, *, #12475, .F. ) ;
#5219=EDGE_LOOP ( 'NONE', ( #8639, #7984, #174, #17028 ) ) ;
#5247=VECTOR ( 'NONE', #14814, 1000.000000000000000 ) ;
#5285=VERTEX_POINT ( 'NONE', #17435 ) ;
#5293=CARTESIAN_POINT ( 'NONE',  ( 0.000000000000000000, 0.000000000000000000, -2.000000000000000000 ) ) ;
#5310=EDGE_CURVE ( 'NONE', #1421, #7830, #14508, .T. ) ;
#5312=CARTESIAN_POINT ( 'NONE',  ( 0.000000000000000000, 0.000000000000000000, -2.000000000000000000 ) ) ;
#5329=ORIENTED_EDGE ( 'NONE', *, *, #13805, .T. ) ;
#5330=EDGE_CURVE ( 'NONE', #1198, #10066, #8966, .T. ) ;
#5333=CARTESIAN_POINT ( 'NONE',  ( 9.458171371211037126, 3.728626979641400219, -2.666481567098320848 ) ) ;
#5344=SURFACE_STYLE_USAGE ( .BOTH. , #12609 ) ;
#5351=EDGE_CURVE ( 'NONE', #9800, #15040, #17670, .T. ) ;
#5379=ORIENTED_EDGE ( 'NONE', *, *, #7811, .F. ) ;
#5433=VERTEX_POINT ( 'NONE', #9401 ) ;
#5437=PRESENTATION_STYLE_ASSIGNMENT (( #5344 ) ) ;
#5438=CARTESIAN_POINT ( 'NONE',  ( 7.374038404635931521, -5.989453865500120600, -2.000000000000000000 ) ) ;
#5443=EDGE_CURVE ( 'NONE', #8628, #11479, #10917, .T. ) ;
#5444=CARTESIAN_POINT ( 'NONE',  ( 0.000000000000000000, 0.000000000000000000, -10.00000000000000000 ) ) ;
#5466=CARTESIAN_POINT ( 'NONE',  ( 0.000000000000000000, 0.000000000000000000, -3.000000000000002665 ) ) ;
#5468=CARTESIAN_POINT ( 'NONE',  ( -10.27627944162877505, 4.200961894323461010, -11.72793873352925331 ) ) ;
#5481=AXIS2_PLACEMENT_3D ( 'NONE', #4657, #12637, #9993 ) ;
#5487=EDGE_LOOP ( 'NONE', ( #4654, #17307, #14687, #14006 ) ) ;
#5497=CARTESIAN_POINT ( 'NONE',  ( -4.281152949374479100, 4.203775615332273397, -1.901951201008075243 ) ) ;
#5504=AXIS2_PLACEMENT_3D ( 'NONE', #16220, #9049, #11845 ) ;
#5508=ADVANCED_FACE ( 'NONE', ( #7235 ), #12576, .T. ) ;
#5509=CIRCLE ( 'NONE', #15663, 9.500000000000001776 ) ;
#5520=FACE_OUTER_BOUND ( 'NONE', #7894, .T. ) ;
#5538=DIRECTION ( 'NONE',  ( 1.224646799147353207E-16, -1.000000000000000000, 0.000000000000000000 ) ) ;
#5543=AXIS2_PLACEMENT_3D ( 'NONE', #1414, #10999, #9646 ) ;
#5566=LINE ( 'NONE', #11084, #16772 ) ;
#5585=DIRECTION ( 'NONE',  ( 1.000000000000000000, 8.881784197001252323E-16, 0.000000000000000000 ) ) ;
#5613=DIRECTION ( 'NONE',  ( 1.000000000000000000, 0.000000000000000000, -0.000000000000000000 ) ) ;
#5620=EDGE_LOOP ( 'NONE', ( #7306, #4544, #7105, #16938 ) ) ;
#5641=DIRECTION ( 'NONE',  ( -1.224646799147353207E-16, 1.000000000000000000, 0.000000000000000000 ) ) ;
#5654=CYLINDRICAL_SURFACE ( 'NONE', #12999, 6.000000000000000888 ) ;
#5681=CARTESIAN_POINT ( 'NONE',  ( 0.000000000000000000, 0.000000000000000000, -2.000000000000000000 ) ) ;
#5690=PLANE ( 'NONE',  #10166 ) ;
#5699=CARTESIAN_POINT ( 'NONE',  ( 0.000000000000000000, 0.000000000000000000, -2.000000000000000000 ) ) ;
#5727=ADVANCED_FACE ( 'NONE', ( #14596 ), #2172, .F. ) ;
#5733=ORIENTED_EDGE ( 'NONE', *, *, #17759, .F. ) ;
#5750=ORIENTED_EDGE ( 'NONE', *, *, #11050, .F. ) ;
#5791=FACE_OUTER_BOUND ( 'NONE', #439, .T. ) ;
#5817=ORIENTED_EDGE ( 'NONE', *, *, #16914, .F. ) ;
#5823=VECTOR ( 'NONE', #1786, 1000.000000000000000 ) ;
#5856=CARTESIAN_POINT ( 'NONE',  ( -8.776279441628885181, -6.799038105676576293, -3.000000000000000888 ) ) ;
#5862=FACE_OUTER_BOUND ( 'NONE', #16136, .T. ) ;
#5876=DIRECTION ( 'NONE',  ( 1.000000000000000000, 0.000000000000000000, 0.000000000000000000 ) ) ;
#5878=CARTESIAN_POINT ( 'NONE',  ( -5.781152949374542160, -1.605699403978851247, -1.901951201008075243 ) ) ;
#5887=CARTESIAN_POINT ( 'NONE',  ( 10.27627944162880702, -4.200961894323389956, -2.000000000000000000 ) ) ;
#5900=ORIENTED_EDGE ( 'NONE', *, *, #4484, .F. ) ;
#5910=CARTESIAN_POINT ( 'NONE',  ( -8.874038404635921751, 3.391377654146875642, -2.000000000000000000 ) ) ;
#5919=EDGE_LOOP ( 'NONE', ( #9185, #7628, #13149, #4915 ) ) ;
#5922=ORIENTED_EDGE ( 'NONE', *, *, #16179, .T. ) ;
#5937=ORIENTED_EDGE ( 'NONE', *, *, #17446, .T. ) ;
#5975=DIRECTION ( 'NONE',  ( -0.5000000000000099920, -0.8660254037844329345, 0.000000000000000000 ) ) ;
#6000=DIRECTION ( 'NONE',  ( 1.000000000000000000, 0.000000000000000000, -0.000000000000000000 ) ) ;
#6006=DIRECTION ( 'NONE',  ( 0.000000000000000000, 0.000000000000000000, -1.000000000000000000 ) ) ;
#6012=AXIS2_PLACEMENT_3D ( 'NONE', #15788, #11600, #6260 ) ;
#6035=LINE ( 'NONE', #7421, #14552 ) ;
#6046=AXIS2_PLACEMENT_3D ( 'NONE', #4918, #8070, #2040 ) ;
#6054=CARTESIAN_POINT ( 'NONE',  ( 0.000000000000000000, 0.000000000000000000, -3.000000000000002665 ) ) ;
#6055=DIRECTION ( 'NONE',  ( -5.026720092345836698E-22, 4.581671729415424240E-22, -1.000000000000000000 ) ) ;
#6063=DIRECTION ( 'NONE',  ( -1.224646799147353207E-16, 1.000000000000000000, 0.000000000000000000 ) ) ;
#6072=EDGE_CURVE ( 'NONE', #4832, #1869, #2309, .T. ) ;
#6088=ORIENTED_EDGE ( 'NONE', *, *, #17358, .T. ) ;
#6094=LINE ( 'NONE', #14551, #10038 ) ;
#6104=CARTESIAN_POINT ( 'NONE',  ( 1.500000000000000666, 5.809475019311125976, -1.901951201008075243 ) ) ;
#6106=CARTESIAN_POINT ( 'NONE',  ( -9.749999999999953815, 3.897114317030088149, -3.000000000000000000 ) ) ;
#6150=ORIENTED_EDGE ( 'NONE', *, *, #8192, .T. ) ;
#6153=CIRCLE ( 'NONE', #2957, 0.9000000000000003553 ) ;
#6159=EDGE_CURVE ( 'NONE', #2839, #7960, #12398, .T. ) ;
#6170=DIRECTION ( 'NONE',  ( 1.000000000000000000, 0.000000000000000000, 0.000000000000000000 ) ) ;
#6172=ADVANCED_FACE ( 'NONE', ( #5862 ), #14217, .F. ) ;
#6205=ADVANCED_FACE ( 'NONE', ( #10214 ), #1809, .T. ) ;
#6223=ORIENTED_EDGE ( 'NONE', *, *, #6159, .F. ) ;
#6237=ORIENTED_EDGE ( 'NONE', *, *, #14569, .T. ) ;
#6260=DIRECTION ( 'NONE',  ( 0.9979201627913403261, -0.06446199418653547619, 0.000000000000000000 ) ) ;
#6267=CARTESIAN_POINT ( 'NONE',  ( 0.000000000000000000, 0.000000000000000000, -3.000000000000000000 ) ) ;
#6268=ORIENTED_EDGE ( 'NONE', *, *, #15189, .T. ) ;
#6269=CARTESIAN_POINT ( 'NONE',  ( 1.746467850512308208E-21, -1.591841644184202181E-21, -6.005572809000082835 ) ) ;
#6272=ORIENTED_EDGE ( 'NONE', *, *, #710, .F. ) ;
#6349=CARTESIAN_POINT ( 'NONE',  ( -7.374038404635891553, 5.989453865500174778, -2.000000000000000000 ) ) ;
#6375=B_SPLINE_CURVE_WITH_KNOTS ( 'NONE', 3,
 ( #15245, #1655, #9610, #1472 ),
 .UNSPECIFIED., .F., .F.,
 ( 4, 4 ),
 ( 0.007932485430080135971, 0.009354825709699440481 ),
 .UNSPECIFIED. ) ;
#6380=PLANE ( 'NONE',  #11317 ) ;
#6388=AXIS2_PLACEMENT_3D ( 'NONE', #13116, #10632, #11655 ) ;
#6390=FACE_OUTER_BOUND ( 'NONE', #11076, .T. ) ;
#6392=B_SPLINE_CURVE_WITH_KNOTS ( 'NONE', 3,
 ( #3775, #3684, #9299, #4765 ),
 .UNSPECIFIED., .F., .F.,
 ( 4, 4 ),
 ( 0.007932485430080137706, 0.009354825709699442216 ),
 .UNSPECIFIED. ) ;
#6397=AXIS2_PLACEMENT_3D ( 'NONE', #14054, #12684, #9681 ) ;
#6398=ORIENTED_EDGE ( 'NONE', *, *, #11670, .F. ) ;
#6400=ORIENTED_EDGE ( 'NONE', *, *, #5443, .T. ) ;
#6419=FACE_OUTER_BOUND ( 'NONE', #3643, .T. ) ;
#6420=STYLED_ITEM ( 'NONE', ( #5437 ), #11123 ) ;
#6425=EDGE_CURVE ( 'NONE', #3366, #10034, #7395, .T. ) ;
#6435=CARTESIAN_POINT ( 'NONE',  ( 1.499999999999999334, -5.809475019311126864, -2.000000000000000000 ) ) ;
#6441=CIRCLE ( 'NONE', #10757, 2.500000000000000000 ) ;
#6455=ORIENTED_EDGE ( 'NONE', *, *, #15879, .F. ) ;
#6456=CIRCLE ( 'NONE', #14271, 10.50000000000000000 ) ;
#6462=ORIENTED_EDGE ( 'NONE', *, *, #2462, .T. ) ;
#6468=FACE_BOUND ( 'NONE', #12862, .T. ) ;
#6482=CARTESIAN_POINT ( 'NONE',  ( -9.166200962222356807, -3.560057785416302689, -2.333128398347827481 ) ) ;
#6536=EDGE_CURVE ( 'NONE', #17313, #11147, #1190, .T. ) ;
#6546=DIRECTION ( 'NONE',  ( -0.000000000000000000, -0.000000000000000000, -1.000000000000000000 ) ) ;
#6554=ORIENTED_EDGE ( 'NONE', *, *, #15595, .F. ) ;
#6572=CARTESIAN_POINT ( 'NONE',  ( 1.500000000000000000, -10.39230484541326405, -3.000000000000000000 ) ) ;
#6575=ORIENTED_EDGE ( 'NONE', *, *, #6849, .T. ) ;
#6618=EDGE_CURVE ( 'NONE', #10285, #17504, #13870, .T. ) ;
#6653=AXIS2_PLACEMENT_3D ( 'NONE', #4749, #8927, #3589 ) ;
#6664=VERTEX_POINT ( 'NONE', #10266 ) ;
#6667=VECTOR ( 'NONE', #15281, 1000.000000000000114 ) ;
#6677=VERTEX_POINT ( 'NONE', #7739 ) ;
#6689=FACE_OUTER_BOUND ( 'NONE', #10611, .T. ) ;
#6716=AXIS2_PLACEMENT_3D ( 'NONE', #11636, #10356, #676 ) ;
#6720=EDGE_CURVE ( 'NONE', #11483, #13130, #17211, .T. ) ;
#6722=CIRCLE ( 'NONE', #12243, 0.9000000000000003553 ) ;
#6726=DIRECTION ( 'NONE',  ( 1.000000000000000000, 0.000000000000000000, 0.000000000000000000 ) ) ;
#6728=ORIENTED_EDGE ( 'NONE', *, *, #8192, .F. ) ;
#6734=AXIS2_PLACEMENT_3D ( 'NONE', #5293, #12460, #15269 ) ;
#6736=CIRCLE ( 'NONE', #1209, 10.50000000000000000 ) ;
#6745=CIRCLE ( 'NONE', #13428, 10.50000000000000000 ) ;
#6760=DIRECTION ( 'NONE',  ( -1.000000000000000000, 0.000000000000000000, 0.000000000000000000 ) ) ;
#6762=AXIS2_PLACEMENT_3D ( 'NONE', #601, #17911, #3600 ) ;
#6771=ORIENTED_EDGE ( 'NONE', *, *, #9109, .T. ) ;
#6777=ORIENTED_EDGE ( 'NONE', *, *, #4107, .F. ) ;
#6802=EDGE_CURVE ( 'NONE', #1572, #729, #4335, .T. ) ;
#6839=CARTESIAN_POINT ( 'NONE',  ( 1.500000000000000666, 5.809475019311125976, -2.000000000000000000 ) ) ;
#6842=DIRECTION ( 'NONE',  ( 0.8660254037844329345, -0.5000000000000099920, 0.000000000000000000 ) ) ;
#6849=EDGE_CURVE ( 'NONE', #14109, #6677, #13309, .T. ) ;
#6856=ORIENTED_EDGE ( 'NONE', *, *, #4191, .F. ) ;
#6857=B_SPLINE_CURVE_WITH_KNOTS ( 'NONE', 3,
 ( #6106, #9106, #9014, #10270 ),
 .UNSPECIFIED., .F., .F.,
 ( 4, 4 ),
 ( 2.843119637709864978E-07, 0.001422633878257846410 ),
 .UNSPECIFIED. ) ;
#6863=DIRECTION ( 'NONE',  ( 0.000000000000000000, 0.000000000000000000, 1.000000000000000000 ) ) ;
#6896=FILL_AREA_STYLE ('',( #13791 ) ) ;
#6902=VECTOR ( 'NONE', #107, 1000.000000000000000 ) ;
#6903=VERTEX_POINT ( 'NONE', #8881 ) ;
#6905=CARTESIAN_POINT ( 'NONE',  ( 5.781152949374518180, -1.605699403978931405, -2.000000000000000000 ) ) ;
#6919=EDGE_LOOP ( 'NONE', ( #11825, #17770, #643, #16034, #16052, #6771, #15361, #15224, #9583, #89, #10076 ) ) ;
#6927=DIRECTION ( 'NONE',  ( 1.000000000000000000, 3.552713678800500929E-15, 0.000000000000000000 ) ) ;
#6959=( GEOMETRIC_REPRESENTATION_CONTEXT ( 3 ) GLOBAL_UNCERTAINTY_ASSIGNED_CONTEXT ( ( #8610 ) ) GLOBAL_UNIT_ASSIGNED_CONTEXT ( ( #13425, #2454, #9749 ) ) REPRESENTATION_CONTEXT ( 'NONE', 'WORKASPACE' ) );
#6973=ORIENTED_EDGE ( 'NONE', *, *, #7540, .F. ) ;
#6976=EDGE_CURVE ( 'NONE', #14024, #9359, #11552, .T. ) ;
#7014=CARTESIAN_POINT ( 'NONE',  ( 0.000000000000000000, 0.000000000000000000, -3.000000000000002665 ) ) ;
#7015=CIRCLE ( 'NONE', #5543, 0.9000000000000003553 ) ;
#7018=ADVANCED_BREP_SHAPE_REPRESENTATION ( '', ( #11123, #3575 ), #15 ) ;
#7034=CARTESIAN_POINT ( 'NONE',  ( 8.250000000000014211, 6.495190528383269601, -3.000000000000000000 ) ) ;
#7037=CARTESIAN_POINT ( 'NONE',  ( -9.500000000000001776, 0.000000000000000000, -2.000000000000000000 ) ) ;
#7041=CONICAL_SURFACE ( 'NONE', #16319, 9.500000000000001776, 0.7853981633974465026 ) ;
#7103=B_SPLINE_CURVE_WITH_KNOTS ( 'NONE', 3,
 ( #7034, #11249, #11535, #10184 ),
 .UNSPECIFIED., .F., .F.,
 ( 4, 4 ),
 ( 2.843119637714455897E-07, 0.001422633878257845976 ),
 .UNSPECIFIED. ) ;
#7105=ORIENTED_EDGE ( 'NONE', *, *, #4484, .T. ) ;
#7110=ORIENTED_EDGE ( 'NONE', *, *, #8996, .F. ) ;
#7113=DIRECTION ( 'NONE',  ( 1.000000000000000000, 0.000000000000000000, 0.000000000000000000 ) ) ;
#7161=DIRECTION ( 'NONE',  ( -1.000000000000000000, 0.000000000000000000, 0.000000000000000000 ) ) ;
#7181=CARTESIAN_POINT ( 'NONE',  ( 4.281152949374508410, -4.203775615332241422, -3.000000000000000888 ) ) ;
#7185=AXIS2_PLACEMENT_3D ( 'NONE', #1308, #10884, #9705 ) ;
#7207=AXIS2_PLACEMENT_3D ( 'NONE', #12658, #69, #2873 ) ;
#7208=AXIS2_PLACEMENT_3D ( 'NONE', #1738, #5975, #11499 ) ;
#7213=ORIENTED_EDGE ( 'NONE', *, *, #7589, .T. ) ;
#7216=DIRECTION ( 'NONE',  ( 0.000000000000000000, 0.000000000000000000, 1.000000000000000000 ) ) ;
#7228=AXIS2_PLACEMENT_3D ( 'NONE', #12033, #3887, #16230 ) ;
#7235=FACE_OUTER_BOUND ( 'NONE', #1187, .T. ) ;
#7243=CARTESIAN_POINT ( 'NONE',  ( 10.27627944162883544, 4.200961894323318013, -11.72793873352922489 ) ) ;
#7266=AXIS2_PLACEMENT_3D ( 'NONE', #7604, #17609, #2083 ) ;
#7268=CARTESIAN_POINT ( 'NONE',  ( -1.500000000000000000, 11.00000000000000000, -9.708203932499369415 ) ) ;
#7283=AXIS2_PLACEMENT_3D ( 'NONE', #13763, #6863, #12394 ) ;
#7306=ORIENTED_EDGE ( 'NONE', *, *, #10158, .F. ) ;
#7366=LINE ( 'NONE', #5887, #13345 ) ;
#7386=CARTESIAN_POINT ( 'NONE',  ( -10.50000000000000000, 0.000000000000000000, -7.794427190999915211 ) ) ;
#7387=LINE ( 'NONE', #9981, #11186 ) ;
#7389=CARTESIAN_POINT ( 'NONE',  ( 0.000000000000000000, 0.000000000000000000, -2.000000000000000000 ) ) ;
#7392=EDGE_CURVE ( 'NONE', #2839, #13145, #9825, .T. ) ;
#7393=CARTESIAN_POINT ( 'NONE',  ( 0.000000000000000000, 0.000000000000000000, -2.000000000000000000 ) ) ;
#7395=LINE ( 'NONE', #12818, #17379 ) ;
#7399=FACE_OUTER_BOUND ( 'NONE', #15267, .T. ) ;
#7402=ORIENTED_EDGE ( 'NONE', *, *, #8369, .F. ) ;
#7407=CARTESIAN_POINT ( 'NONE',  ( 4.281152949374537720, 4.203775615332211224, -2.000000000000000000 ) ) ;
#7409=DIRECTION ( 'NONE',  ( -0.000000000000000000, -0.000000000000000000, -1.000000000000000000 ) ) ;
#7421=CARTESIAN_POINT ( 'NONE',  ( -8.776279441628744848, 6.799038105676760146, -3.000000000000000888 ) ) ;
#7424=DIRECTION ( 'NONE',  ( -1.000000000000000000, 0.000000000000000000, 0.000000000000000000 ) ) ;
#7432=DIRECTION ( 'NONE',  ( -0.8660254037844397068, -0.4999999999999981126, 0.000000000000000000 ) ) ;
#7436=CARTESIAN_POINT ( 'NONE',  ( 10.50000000000000000, 1.285879139104720831E-15, -6.005572809000082835 ) ) ;
#7459=AXIS2_PLACEMENT_3D ( 'NONE', #7389, #12903, #12159 ) ;
#7463=DIRECTION ( 'NONE',  ( 5.026720092345836698E-22, -4.581671729415424240E-22, 1.000000000000000000 ) ) ;
#7471=DIRECTION ( 'NONE',  ( -5.026720092345836698E-22, 4.581671729415424240E-22, -1.000000000000000000 ) ) ;
#7484=CARTESIAN_POINT ( 'NONE',  ( -6.000000000000000888, 0.000000000000000000, -2.000000000000000000 ) ) ;
#7503=DIRECTION ( 'NONE',  ( -0.8660254037844329345, 0.5000000000000099920, 0.000000000000000000 ) ) ;
#7518=ORIENTED_EDGE ( 'NONE', *, *, #14055, .F. ) ;
#7534=ORIENTED_EDGE ( 'NONE', *, *, #16958, .T. ) ;
#7540=EDGE_CURVE ( 'NONE', #13908, #15040, #6392, .T. ) ;
#7566=LINE ( 'NONE', #3388, #12746 ) ;
#7567=CARTESIAN_POINT ( 'NONE',  ( -1.500000000000000000, -11.00000000000000000, -3.000000000000000000 ) ) ;
#7568=ORIENTED_EDGE ( 'NONE', *, *, #4788, .F. ) ;
#7572=CARTESIAN_POINT ( 'NONE',  ( -1.500000000000000000, 11.00000000000000000, -2.000000000000000000 ) ) ;
#7588=VERTEX_POINT ( 'NONE', #6839 ) ;
#7589=EDGE_CURVE ( 'NONE', #6677, #1421, #11863, .T. ) ;
#7598=CARTESIAN_POINT ( 'NONE',  ( -5.781152949374509298, 1.605699403978973372, -2.000000000000000000 ) ) ;
#7604=CARTESIAN_POINT ( 'NONE',  ( 0.000000000000000000, 0.000000000000000000, -2.000000000000000000 ) ) ;
#7616=CARTESIAN_POINT ( 'NONE',  ( 4.281152949374507521, -4.203775615332241422, -1.901951201008075243 ) ) ;
#7626=SURFACE_STYLE_FILL_AREA ( #2280 ) ;
#7628=ORIENTED_EDGE ( 'NONE', *, *, #137, .T. ) ;
#7635=ORIENTED_EDGE ( 'NONE', *, *, #16853, .F. ) ;
#7645=ORIENTED_EDGE ( 'NONE', *, *, #15322, .T. ) ;
#7686=DIRECTION ( 'NONE',  ( 0.000000000000000000, 0.000000000000000000, -1.000000000000000000 ) ) ;
#7739=CARTESIAN_POINT ( 'NONE',  ( -9.750000000000035527, -3.897114317029883868, -3.000000000000002665 ) ) ;
#7782=AXIS2_PLACEMENT_3D ( 'NONE', #10296, #7686, #2346 ) ;
#7806=AXIS2_PLACEMENT_3D ( 'NONE', #5681, #12671, #7161 ) ;
#7811=EDGE_CURVE ( 'NONE', #13145, #5285, #10084, .T. ) ;
#7814=ADVANCED_FACE ( 'NONE', ( #7399 ), #14285, .F. ) ;
#7830=VERTEX_POINT ( 'NONE', #415 ) ;
#7834=EDGE_CURVE ( 'NONE', #625, #9800, #7103, .T. ) ;
#7835=DIRECTION ( 'NONE',  ( 0.000000000000000000, 0.000000000000000000, -1.000000000000000000 ) ) ;
#7861=DIRECTION ( 'NONE',  ( -0.8660254037844363761, 0.5000000000000038858, 0.000000000000000000 ) ) ;
#7889=DIRECTION ( 'NONE',  ( 1.000000000000000000, 1.776356839400250465E-15, 0.000000000000000000 ) ) ;
#7894=EDGE_LOOP ( 'NONE', ( #10062, #14436, #17532, #1049 ) ) ;
#7897=CARTESIAN_POINT ( 'NONE',  ( -7.666200962222251114, 6.158133996769793228, -2.333128398347828369 ) ) ;
#7906=DIRECTION ( 'NONE',  ( 5.026720092345836698E-22, -4.581671729415424240E-22, 1.000000000000000000 ) ) ;
#7909=DIRECTION ( 'NONE',  ( 1.000000000000000000, 0.000000000000000000, 0.000000000000000000 ) ) ;
#7943=EDGE_CURVE ( 'NONE', #15452, #3773, #6857, .T. ) ;
#7959=ADVANCED_FACE ( 'NONE', ( #13186, #4827 ), #14565, .F. ) ;
#7960=VERTEX_POINT ( 'NONE', #764 ) ;
#7984=ORIENTED_EDGE ( 'NONE', *, *, #2645, .T. ) ;
#7987=LINE ( 'NONE', #16426, #3811 ) ;
#8020=CARTESIAN_POINT ( 'NONE',  ( -10.47816170930907553, 0.6768509389586230274, -6.005572809000082835 ) ) ;
#8023=ADVANCED_FACE ( 'NONE', ( #16320 ), #9482, .F. ) ;
#8039=ORIENTED_EDGE ( 'NONE', *, *, #1700, .F. ) ;
#8043=DIRECTION ( 'NONE',  ( 0.000000000000000000, 0.000000000000000000, 1.000000000000000000 ) ) ;
#8045=ORIENTED_EDGE ( 'NONE', *, *, #8272, .F. ) ;
#8051=CARTESIAN_POINT ( 'NONE',  ( 4.281152949374505745, -4.203775615332239646, -2.000000000000000000 ) ) ;
#8070=DIRECTION ( 'NONE',  ( 0.000000000000000000, 0.000000000000000000, 1.000000000000000000 ) ) ;
#8075=EDGE_CURVE ( 'NONE', #9144, #14530, #9887, .T. ) ;
#8098=VECTOR ( 'NONE', #6006, 1000.000000000000000 ) ;
#8184=VECTOR ( 'NONE', #16175, 1000.000000000000000 ) ;
#8192=EDGE_CURVE ( 'NONE', #12819, #16631, #6153, .T. ) ;
#8219=LINE ( 'NONE', #14021, #4295 ) ;
#8222=EDGE_LOOP ( 'NONE', ( #10404, #5733, #10372, #6973 ) ) ;
#8227=CARTESIAN_POINT ( 'NONE',  ( -5.781152949374509298, 1.605699403978974260, -1.901951201008075243 ) ) ;
#8235=B_SPLINE_CURVE_WITH_KNOTS ( 'NONE', 3,
 ( #17635, #819, #7897, #6349 ),
 .UNSPECIFIED., .F., .F.,
 ( 4, 4 ),
 ( 2.843119637691541009E-07, 0.001422633878257847928 ),
 .UNSPECIFIED. ) ;
#8237=DIRECTION ( 'NONE',  ( 0.8660254037844328234, -0.5000000000000099920, 0.000000000000000000 ) ) ;
#8244=ORIENTED_EDGE ( 'NONE', *, *, #5099, .F. ) ;
#8254=CARTESIAN_POINT ( 'NONE',  ( 0.000000000000000000, 0.000000000000000000, -10.00000000000000000 ) ) ;
#8257=ORIENTED_EDGE ( 'NONE', *, *, #16240, .F. ) ;
#8261=CARTESIAN_POINT ( 'NONE',  ( 0.000000000000000000, 0.000000000000000000, -3.000000000000002665 ) ) ;
#8265=ORIENTED_EDGE ( 'NONE', *, *, #8718, .F. ) ;
#8272=EDGE_CURVE ( 'NONE', #11446, #9144, #13744, .T. ) ;
#8275=DIRECTION ( 'NONE',  ( 0.000000000000000000, 0.000000000000000000, -1.000000000000000000 ) ) ;
#8282=CARTESIAN_POINT ( 'NONE',  ( -5.781152949374509298, 1.605699403978974260, -3.000000000000000888 ) ) ;
#8292=ADVANCED_FACE ( 'NONE', ( #4499 ), #7041, .T. ) ;
#8302=ORIENTED_EDGE ( 'NONE', *, *, #4069, .T. ) ;
#8316=CIRCLE ( 'NONE', #7185, 6.000000000000000888 ) ;
#8322=DIRECTION ( 'NONE',  ( 0.000000000000000000, 0.000000000000000000, 1.000000000000000000 ) ) ;
#8331=DIRECTION ( 'NONE',  ( -1.224646799147353207E-16, 1.000000000000000000, 0.000000000000000000 ) ) ;
#8365=ORIENTED_EDGE ( 'NONE', *, *, #17857, .T. ) ;
#8369=EDGE_CURVE ( 'NONE', #13928, #2781, #14390, .T. ) ;
#8377=ORIENTED_EDGE ( 'NONE', *, *, #8075, .T. ) ;
#8413=CONICAL_SURFACE ( 'NONE', #7266, 9.500000000000001776, 0.7853981633974465026 ) ;
#8417=ORIENTED_EDGE ( 'NONE', *, *, #16179, .F. ) ;
#8459=ADVANCED_FACE ( 'NONE', ( #14484 ), #9204, .F. ) ;
#8477=DIRECTION ( 'NONE',  ( 1.000000000000000000, 0.000000000000000000, 0.000000000000000000 ) ) ;
#8482=DIRECTION ( 'NONE',  ( -1.000000000000000000, 0.000000000000000000, 0.000000000000000000 ) ) ;
#8494=CARTESIAN_POINT ( 'NONE',  ( -1.500000000000000666, -5.809475019311125976, -3.000000000000000000 ) ) ;
#8526=ORIENTED_EDGE ( 'NONE', *, *, #16853, .T. ) ;
#8533=DIRECTION ( 'NONE',  ( 0.000000000000000000, 0.000000000000000000, 1.000000000000000000 ) ) ;
#8544=EDGE_LOOP ( 'NONE', ( #11945, #5104, #6728, #3160, #4739 ) ) ;
#8569=CARTESIAN_POINT ( 'NONE',  ( 1.746467850512308208E-21, -1.591841644184202181E-21, -6.005572809000082835 ) ) ;
#8582=DIRECTION ( 'NONE',  ( 1.000000000000000000, 1.776356839400250465E-15, 0.000000000000000000 ) ) ;
#8610=UNCERTAINTY_MEASURE_WITH_UNIT (LENGTH_MEASURE( 1.000000000000000082E-05 ), #13425, 'distance_accuracy_value', 'NONE');
#8616=FACE_OUTER_BOUND ( 'NONE', #17476, .T. ) ;
#8619=CIRCLE ( 'NONE', #16723, 10.50000000000000000 ) ;
#8628=VERTEX_POINT ( 'NONE', #7598 ) ;
#8631=VECTOR ( 'NONE', #11763, 1000.000000000000000 ) ;
#8632=CARTESIAN_POINT ( 'NONE',  ( 10.50000000000000000, 1.285879139104720831E-15, -10.00000000000000000 ) ) ;
#8639=ORIENTED_EDGE ( 'NONE', *, *, #15322, .F. ) ;
#8646=B_SPLINE_CURVE_WITH_KNOTS ( 'NONE', 3,
 ( #12507, #13454, #5092, #10697 ),
 .UNSPECIFIED., .F., .F.,
 ( 4, 4 ),
 ( 2.843119637691541009E-07, 0.001422633878257849012 ),
 .UNSPECIFIED. ) ;
#8654=CIRCLE ( 'NONE', #9779, 9.500000000000001776 ) ;
#8655=ORIENTED_EDGE ( 'NONE', *, *, #17282, .T. ) ;
#8688=DIRECTION ( 'NONE',  ( -0.4999999999999981126, 0.8660254037844397068, 0.000000000000000000 ) ) ;
#8718=EDGE_CURVE ( 'NONE', #1869, #13908, #6745, .T. ) ;
#8735=CARTESIAN_POINT ( 'NONE',  ( -10.27627944162877505, 4.200961894323461010, -3.000000000000000888 ) ) ;
#8790=AXIS2_PLACEMENT_3D ( 'NONE', #14696, #11961, #11866 ) ;
#8825=FACE_OUTER_BOUND ( 'NONE', #9055, .T. ) ;
#8834=ORIENTED_EDGE ( 'NONE', *, *, #13382, .F. ) ;
#8857=ORIENTED_EDGE ( 'NONE', *, *, #6849, .F. ) ;
#8881=CARTESIAN_POINT ( 'NONE',  ( 2.500000000000000000, 0.000000000000000000, -10.00000000000000000 ) ) ;
#8882=ADVANCED_FACE ( 'NONE', ( #4883 ), #9912, .F. ) ;
#8885=CARTESIAN_POINT ( 'NONE',  ( -2.500000000000000000, 3.061616997868383141E-16, -3.000000000000000000 ) ) ;
#8895=CARTESIAN_POINT ( 'NONE',  ( 0.000000000000000000, 0.000000000000000000, -3.000000000000000000 ) ) ;
#8899=ORIENTED_EDGE ( 'NONE', *, *, #6159, .T. ) ;
#8911=CARTESIAN_POINT ( 'NONE',  ( 1.746467850512308208E-21, -1.591841644184202181E-21, -6.005572809000082835 ) ) ;
#8927=DIRECTION ( 'NONE',  ( 0.000000000000000000, 0.000000000000000000, 1.000000000000000000 ) ) ;
#8932=CARTESIAN_POINT ( 'NONE',  ( -7.666200962222379900, -6.158133996769632468, -2.333128398347828369 ) ) ;
#8939=ORIENTED_EDGE ( 'NONE', *, *, #12774, .F. ) ;
#8959=VERTEX_POINT ( 'NONE', #15213 ) ;
#8966=LINE ( 'NONE', #7616, #8631 ) ;
#8972=AXIS2_PLACEMENT_3D ( 'NONE', #11034, #10856, #10941 ) ;
#8996=EDGE_CURVE ( 'NONE', #3773, #8628, #2529, .T. ) ;
#8998=VECTOR ( 'NONE', #10772, 1000.000000000000000 ) ;
#9005=CONICAL_SURFACE ( 'NONE', #1192, 9.500000000000001776, 0.7853981633974465026 ) ;
#9014=CARTESIAN_POINT ( 'NONE',  ( -9.166200962222282200, 3.560057785416494980, -2.333128398347827037 ) ) ;
#9037=DIRECTION ( 'NONE',  ( 0.000000000000000000, 0.000000000000000000, -1.000000000000000000 ) ) ;
#9049=DIRECTION ( 'NONE',  ( -5.026720092345836698E-22, 4.581671729415424240E-22, -1.000000000000000000 ) ) ;
#9055=EDGE_LOOP ( 'NONE', ( #14830, #12593, #14899, #11421 ) ) ;
#9066=TOROIDAL_SURFACE ( 'NONE', #1843, 10.40000000000000036, 0.9000000000000003553 ) ;
#9080=AXIS2_PLACEMENT_3D ( 'NONE', #11579, #14507, #10306 ) ;
#9084=ORIENTED_EDGE ( 'NONE', *, *, #12401, .T. ) ;
#9097=ADVANCED_FACE ( 'NONE', ( #15763 ), #15436, .T. ) ;
#9102=ORIENTED_EDGE ( 'NONE', *, *, #7589, .F. ) ;
#9106=CARTESIAN_POINT ( 'NONE',  ( -9.458171371210985612, 3.728626979641533001, -2.666481567098319072 ) ) ;
#9109=EDGE_CURVE ( 'NONE', #1421, #15452, #1849, .T. ) ;
#9144=VERTEX_POINT ( 'NONE', #14316 ) ;
#9185=ORIENTED_EDGE ( 'NONE', *, *, #17282, .F. ) ;
#9204=PLANE ( 'NONE',  #3857 ) ;
#9238=FILL_AREA_STYLE_COLOUR ( '', #11583 ) ;
#9246=AXIS2_PLACEMENT_3D ( 'NONE', #13277, #13106, #17112 ) ;
#9251=CARTESIAN_POINT ( 'NONE',  ( 2.500000000000000000, 0.000000000000000000, -3.000000000000000000 ) ) ;
#9272=DIRECTION ( 'NONE',  ( 1.000000000000000000, 0.000000000000000000, 0.000000000000000000 ) ) ;
#9299=CARTESIAN_POINT ( 'NONE',  ( 1.500000000000000222, 9.718191103688258892, -2.333127728361106712 ) ) ;
#9312=AXIS2_PLACEMENT_3D ( 'NONE', #851, #7835, #2319 ) ;
#9334=AXIS2_PLACEMENT_3D ( 'NONE', #12820, #11441, #17007 ) ;
#9354=EDGE_CURVE ( 'NONE', #14350, #14070, #4859, .T. ) ;
#9359=VERTEX_POINT ( 'NONE', #5123 ) ;
#9401=CARTESIAN_POINT ( 'NONE',  ( 10.47816170930907553, -0.6768509389586216951, -7.794427190999915211 ) ) ;
#9418=ORIENTED_EDGE ( 'NONE', *, *, #8369, .T. ) ;
#9428=ADVANCED_FACE ( 'NONE', ( #3422 ), #10297, .T. ) ;
#9464=FACE_OUTER_BOUND ( 'NONE', #12194, .T. ) ;
#9482=PLANE ( 'NONE',  #13676 ) ;
#9507=FACE_OUTER_BOUND ( 'NONE', #11969, .T. ) ;
#9543=CARTESIAN_POINT ( 'NONE',  ( 9.750000000000010658, 3.897114317029950037, -3.000000000000002665 ) ) ;
#9551=CIRCLE ( 'NONE', #6388, 6.000000000000000888 ) ;
#9567=CARTESIAN_POINT ( 'NONE',  ( 0.000000000000000000, 0.000000000000000000, -2.000000000000000000 ) ) ;
#9579=VECTOR ( 'NONE', #16948, 1000.000000000000000 ) ;
#9583=ORIENTED_EDGE ( 'NONE', *, *, #8718, .T. ) ;
#9610=CARTESIAN_POINT ( 'NONE',  ( -1.499999999999999778, 9.718191103688258892, -2.333127728361106268 ) ) ;
#9612=EDGE_LOOP ( 'NONE', ( #6398, #10236, #15484, #15557, #10446 ) ) ;
#9637=DIRECTION ( 'NONE',  ( 0.000000000000000000, 0.000000000000000000, -1.000000000000000000 ) ) ;
#9646=DIRECTION ( 'NONE',  ( -0.9979201627913403261, 0.06446199418653535129, 0.000000000000000000 ) ) ;
#9652=EDGE_LOOP ( 'NONE', ( #7518, #6777, #5900, #13705 ) ) ;
#9657=DIRECTION ( 'NONE',  ( -5.026720092345836698E-22, 4.581671729415424240E-22, -1.000000000000000000 ) ) ;
#9681=DIRECTION ( 'NONE',  ( -1.000000000000000000, 0.000000000000000000, 0.000000000000000000 ) ) ;
#9690=CARTESIAN_POINT ( 'NONE',  ( 8.874038404635971489, 3.391377654146752629, -2.000000000000000000 ) ) ;
#9695=CARTESIAN_POINT ( 'NONE',  ( 0.000000000000000000, 0.000000000000000000, -3.000000000000000000 ) ) ;
#9696=DIRECTION ( 'NONE',  ( 1.000000000000000000, 0.000000000000000000, 0.000000000000000000 ) ) ;
#9705=DIRECTION ( 'NONE',  ( 1.000000000000000000, 0.000000000000000000, 0.000000000000000000 ) ) ;
#9713=CARTESIAN_POINT ( 'NONE',  ( 9.480241546517731877, -0.6123889447720862744, -6.899999999999998579 ) ) ;
#9718=PLANE ( 'NONE',  #6734 ) ;
#9727=DIRECTION ( 'NONE',  ( 0.000000000000000000, 0.000000000000000000, -1.000000000000000000 ) ) ;
#9736=ORIENTED_EDGE ( 'NONE', *, *, #4639, .T. ) ;
#9749=( NAMED_UNIT ( * ) SI_UNIT ( $, .STERADIAN. ) SOLID_ANGLE_UNIT ( ) );
#9753=CYLINDRICAL_SURFACE ( 'NONE', #7806, 10.50000000000000000 ) ;
#9755=ORIENTED_EDGE ( 'NONE', *, *, #6976, .T. ) ;
#9779=AXIS2_PLACEMENT_3D ( 'NONE', #359, #8322, #2987 ) ;
#9792=VERTEX_POINT ( 'NONE', #17208 ) ;
#9800=VERTEX_POINT ( 'NONE', #3758 ) ;
#9819=DIRECTION ( 'NONE',  ( -0.8660254037844432595, -0.4999999999999921174, 0.000000000000000000 ) ) ;
#9820=EDGE_CURVE ( 'NONE', #3773, #12766, #14489, .T. ) ;
#9825=CIRCLE ( 'NONE', #15049, 6.000000000000000888 ) ;
#9826=VERTEX_POINT ( 'NONE', #11726 ) ;
#9829=ORIENTED_EDGE ( 'NONE', *, *, #13419, .T. ) ;
#9832=DIRECTION ( 'NONE',  ( 0.9979201627913403261, -0.06446199418653547619, 0.000000000000000000 ) ) ;
#9839=CARTESIAN_POINT ( 'NONE',  ( -9.500000000000001776, 0.000000000000000000, -2.000000000000000000 ) ) ;
#9846=ORIENTED_EDGE ( 'NONE', *, *, #4147, .F. ) ;
#9886=FACE_OUTER_BOUND ( 'NONE', #5919, .T. ) ;
#9887=CIRCLE ( 'NONE', #11932, 9.500000000000001776 ) ;
#9892=CARTESIAN_POINT ( 'NONE',  ( 0.000000000000000000, 0.000000000000000000, -3.000000000000002665 ) ) ;
#9912=TOROIDAL_SURFACE ( 'NONE', #8790, 10.40000000000000036, 0.9000000000000003553 ) ;
#9935=CARTESIAN_POINT ( 'NONE',  ( 0.000000000000000000, 0.000000000000000000, -1.901951201008075243 ) ) ;
#9960=DIRECTION ( 'NONE',  ( -0.8660254037844363761, 0.5000000000000038858, 0.000000000000000000 ) ) ;
#9972=ORIENTED_EDGE ( 'NONE', *, *, #17857, .F. ) ;
#9981=CARTESIAN_POINT ( 'NONE',  ( 8.776279441628796363, -6.799038105676699750, -2.000000000000000000 ) ) ;
#9986=ORIENTED_EDGE ( 'NONE', *, *, #12922, .T. ) ;
#9991=ORIENTED_EDGE ( 'NONE', *, *, #6618, .F. ) ;
#9993=DIRECTION ( 'NONE',  ( -1.000000000000000000, 0.000000000000000000, 0.000000000000000000 ) ) ;
#10008=ORIENTED_EDGE ( 'NONE', *, *, #6072, .F. ) ;
#10034=VERTEX_POINT ( 'NONE', #467 ) ;
#10038=VECTOR ( 'NONE', #4735, 1000.000000000000000 ) ;
#10043=DIRECTION ( 'NONE',  ( 1.000000000000000000, 0.000000000000000000, 0.000000000000000000 ) ) ;
#10060=ORIENTED_EDGE ( 'NONE', *, *, #10958, .F. ) ;
#10062=ORIENTED_EDGE ( 'NONE', *, *, #14569, .F. ) ;
#10064=CARTESIAN_POINT ( 'NONE',  ( 0.000000000000000000, 0.000000000000000000, -1.901951201008075243 ) ) ;
#10066=VERTEX_POINT ( 'NONE', #7181 ) ;
#10076=ORIENTED_EDGE ( 'NONE', *, *, #10556, .T. ) ;
#10079=ADVANCED_FACE ( 'NONE', ( #10240 ), #11311, .T. ) ;
#10084=LINE ( 'NONE', #15636, #8098 ) ;
#10094=CARTESIAN_POINT ( 'NONE',  ( 0.000000000000000000, 0.000000000000000000, -2.000000000000000000 ) ) ;
#10098=CARTESIAN_POINT ( 'NONE',  ( 0.000000000000000000, 0.000000000000000000, -10.00000000000000000 ) ) ;
#10119=ORIENTED_EDGE ( 'NONE', *, *, #2231, .F. ) ;
#10134=STYLED_ITEM ( 'NONE', ( #14519 ), #7018 ) ;
#10148=VECTOR ( 'NONE', #11683, 1000.000000000000000 ) ;
#10158=EDGE_CURVE ( 'NONE', #8959, #729, #7366, .T. ) ;
#10160=ADVANCED_FACE ( 'NONE', ( #3362 ), #15510, .F. ) ;
#10166=AXIS2_PLACEMENT_3D ( 'NONE', #12414, #12509, #8331 ) ;
#10177=CARTESIAN_POINT ( 'NONE',  ( 5.781152949374519956, -1.605699403978931850, -3.000000000000000888 ) ) ;
#10178=DIRECTION ( 'NONE',  ( -0.000000000000000000, -0.000000000000000000, -1.000000000000000000 ) ) ;
#10184=CARTESIAN_POINT ( 'NONE',  ( 7.374038404635976818, 5.989453865500072638, -2.000000000000000000 ) ) ;
#10200=ORIENTED_EDGE ( 'NONE', *, *, #10647, .F. ) ;
#10206=DIRECTION ( 'NONE',  ( -0.06446199418653550395, -0.9979201627913403261, -4.248110196704583871E-22 ) ) ;
#10207=ORIENTED_EDGE ( 'NONE', *, *, #17843, .T. ) ;
#10214=FACE_OUTER_BOUND ( 'NONE', #9652, .T. ) ;
#10215=CARTESIAN_POINT ( 'NONE',  ( 0.000000000000000000, 0.000000000000000000, -3.000000000000002665 ) ) ;
#10231=CARTESIAN_POINT ( 'NONE',  ( 0.000000000000000000, 0.000000000000000000, -3.000000000000000000 ) ) ;
#10235=EDGE_CURVE ( 'NONE', #14350, #12819, #20, .T. ) ;
#10236=ORIENTED_EDGE ( 'NONE', *, *, #12774, .T. ) ;
#10239=CIRCLE ( 'NONE', #12854, 10.50000000000000000 ) ;
#10240=FACE_OUTER_BOUND ( 'NONE', #1288, .T. ) ;
#10246=ORIENTED_EDGE ( 'NONE', *, *, #14726, .T. ) ;
#10252=ADVANCED_FACE ( 'NONE', ( #6419 ), #8413, .T. ) ;
#10266=CARTESIAN_POINT ( 'NONE',  ( 8.249999999999971578, -6.495190528383328221, -3.000000000000002665 ) ) ;
#10270=CARTESIAN_POINT ( 'NONE',  ( -8.874038404635921751, 3.391377654146875642, -2.000000000000000000 ) ) ;
#10285=VERTEX_POINT ( 'NONE', #4955 ) ;
#10296=CARTESIAN_POINT ( 'NONE',  ( 0.000000000000000000, 0.000000000000000000, -1.901951201008075243 ) ) ;
#10297=PLANE ( 'NONE',  #15922 ) ;
#10306=DIRECTION ( 'NONE',  ( 1.000000000000000000, 0.000000000000000000, 0.000000000000000000 ) ) ;
#10312=DIRECTION ( 'NONE',  ( 0.000000000000000000, 0.000000000000000000, 1.000000000000000000 ) ) ;
#10356=DIRECTION ( 'NONE',  ( 0.000000000000000000, 0.000000000000000000, 1.000000000000000000 ) ) ;
#10359=EDGE_CURVE ( 'NONE', #10285, #11171, #17946, .T. ) ;
#10368=AXIS2_PLACEMENT_3D ( 'NONE', #10098, #688, #13012 ) ;
#10372=ORIENTED_EDGE ( 'NONE', *, *, #2220, .F. ) ;
#10404=ORIENTED_EDGE ( 'NONE', *, *, #2109, .F. ) ;
#10414=ORIENTED_EDGE ( 'NONE', *, *, #16354, .F. ) ;
#10418=ORIENTED_EDGE ( 'NONE', *, *, #10531, .T. ) ;
#10432=CLOSED_SHELL ( 'NONE', ( #3367, #8882, #15490, #3802, #1936, #1600, #2076, #13715, #4738, #15899, #1240, #10933, #13157, #2308, #8292, #9097, #915, #14698, #10252, #5727, #13864, #6172, #388, #7814, #4734, #12210, #15925, #14128, #13975, #7959, #14536, #9428, #10160, #6205, #8023, #5508, #15826, #12335, #12930, #10079, #8459, #2988, #15848, #1668 ) ) ;
#10446=ORIENTED_EDGE ( 'NONE', *, *, #1996, .T. ) ;
#10449=LINE ( 'NONE', #5856, #13077 ) ;
#10471=ORIENTED_EDGE ( 'NONE', *, *, #10958, .T. ) ;
#10473=CIRCLE ( 'NONE', #3540, 10.50000000000000000 ) ;
#10491=ORIENTED_EDGE ( 'NONE', *, *, #4788, .T. ) ;
#10510=ORIENTED_EDGE ( 'NONE', *, *, #7834, .F. ) ;
#10523=DIRECTION ( 'NONE',  ( -0.9979201627913402151, 0.06446199418653550395, 5.311609029246448998E-22 ) ) ;
#10531=EDGE_CURVE ( 'NONE', #4832, #14580, #8235, .T. ) ;
#10556=EDGE_CURVE ( 'NONE', #625, #11483, #11896, .T. ) ;
#10558=CARTESIAN_POINT ( 'NONE',  ( -1.500000000000000222, -9.380831519646861238, -2.000000000000000000 ) ) ;
#10582=CARTESIAN_POINT ( 'NONE',  ( 0.000000000000000000, 0.000000000000000000, -3.000000000000002665 ) ) ;
#10590=CARTESIAN_POINT ( 'NONE',  ( 0.000000000000000000, 0.000000000000000000, -3.000000000000002665 ) ) ;
#10611=EDGE_LOOP ( 'NONE', ( #5195, #7534, #13407, #8039, #8834 ) ) ;
#10619=CARTESIAN_POINT ( 'NONE',  ( -8.874038404635992805, -3.391377654146690013, -2.000000000000000000 ) ) ;
#10632=DIRECTION ( 'NONE',  ( 0.000000000000000000, 0.000000000000000000, 1.000000000000000000 ) ) ;
#10647=EDGE_CURVE ( 'NONE', #11147, #17504, #3759, .T. ) ;
#10656=EDGE_LOOP ( 'NONE', ( #14287, #1350, #9418, #11008 ) ) ;
#10686=LINE ( 'NONE', #17826, #3971 ) ;
#10697=CARTESIAN_POINT ( 'NONE',  ( 8.874038404635943067, -3.391377654146811693, -2.000000000000000000 ) ) ;
#10757=AXIS2_PLACEMENT_3D ( 'NONE', #13011, #14656, #504 ) ;
#10772=DIRECTION ( 'NONE',  ( 0.000000000000000000, 0.000000000000000000, -1.000000000000000000 ) ) ;
#10814=LINE ( 'NONE', #7037, #2129 ) ;
#10816=ORIENTED_EDGE ( 'NONE', *, *, #15595, .T. ) ;
#10821=EDGE_CURVE ( 'NONE', #12450, #17480, #4379, .T. ) ;
#10832=ORIENTED_EDGE ( 'NONE', *, *, #13233, .F. ) ;
#10837=ORIENTED_EDGE ( 'NONE', *, *, #7392, .F. ) ;
#10844=DIRECTION ( 'NONE',  ( 1.000000000000000000, 0.000000000000000000, -0.000000000000000000 ) ) ;
#10856=DIRECTION ( 'NONE',  ( -0.000000000000000000, -0.000000000000000000, -1.000000000000000000 ) ) ;
#10861=FACE_OUTER_BOUND ( 'NONE', #5219, .T. ) ;
#10866=CARTESIAN_POINT ( 'NONE',  ( -7.374038404635891553, 5.989453865500174778, -2.000000000000000000 ) ) ;
#10870=EDGE_CURVE ( 'NONE', #11479, #15452, #14546, .T. ) ;
#10884=DIRECTION ( 'NONE',  ( -0.000000000000000000, -0.000000000000000000, -1.000000000000000000 ) ) ;
#10905=AXIS2_PLACEMENT_3D ( 'NONE', #7014, #8275, #1392 ) ;
#10917=LINE ( 'NONE', #8227, #2852 ) ;
#10932=AXIS2_PLACEMENT_3D ( 'NONE', #9567, #13672, #4056 ) ;
#10933=ADVANCED_FACE ( 'NONE', ( #8825 ), #1757, .T. ) ;
#10934=CARTESIAN_POINT ( 'NONE',  ( -1.500000000000000222, -9.380831519646861238, -2.000000000000000000 ) ) ;
#10937=EDGE_LOOP ( 'NONE', ( #13943, #17147, #16707, #4017, #11778 ) ) ;
#10941=DIRECTION ( 'NONE',  ( 1.000000000000000000, 0.000000000000000000, 0.000000000000000000 ) ) ;
#10945=DIRECTION ( 'NONE',  ( -1.000000000000000000, 0.000000000000000000, 0.000000000000000000 ) ) ;
#10958=EDGE_CURVE ( 'NONE', #10034, #13969, #14549, .T. ) ;
#10989=FACE_OUTER_BOUND ( 'NONE', #1851, .T. ) ;
#10999=DIRECTION ( 'NONE',  ( 0.06446199418653537905, 0.9979201627913403261, 4.248110196704583871E-22 ) ) ;
#11008=ORIENTED_EDGE ( 'NONE', *, *, #480, .T. ) ;
#11020=DIRECTION ( 'NONE',  ( 0.000000000000000000, 0.000000000000000000, -1.000000000000000000 ) ) ;
#11034=CARTESIAN_POINT ( 'NONE',  ( 0.000000000000000000, 0.000000000000000000, -2.000000000000000000 ) ) ;
#11038=CYLINDRICAL_SURFACE ( 'NONE', #6397, 6.000000000000000888 ) ;
#11050=EDGE_CURVE ( 'NONE', #6664, #11446, #2099, .T. ) ;
#11076=EDGE_LOOP ( 'NONE', ( #2421, #8302, #318, #3577, #6088, #16344, #6575, #7213, #3344, #4048, #15498 ) ) ;
#11084=CARTESIAN_POINT ( 'NONE',  ( -10.27627944162886209, -4.200961894323246071, -3.000000000000000888 ) ) ;
#11109=EDGE_LOOP ( 'NONE', ( #8526, #7645 ) ) ;
#11123=MANIFOLD_SOLID_BREP ( 'Cavity1', #10432 ) ;
#11128=( NAMED_UNIT ( * ) PLANE_ANGLE_UNIT ( ) SI_UNIT ( $, .RADIAN. ) );
#11136=CARTESIAN_POINT ( 'NONE',  ( 0.000000000000000000, 0.000000000000000000, -2.000000000000000000 ) ) ;
#11147=VERTEX_POINT ( 'NONE', #1290 ) ;
#11157=ORIENTED_EDGE ( 'NONE', *, *, #9820, .T. ) ;
#11166=CARTESIAN_POINT ( 'NONE',  ( 0.000000000000000000, 0.000000000000000000, -1.901951201008075243 ) ) ;
#11171=VERTEX_POINT ( 'NONE', #9 ) ;
#11175=CARTESIAN_POINT ( 'NONE',  ( 0.000000000000000000, 0.000000000000000000, -2.000000000000000000 ) ) ;
#11186=VECTOR ( 'NONE', #12901, 999.9999999999998863 ) ;
#11216=DIRECTION ( 'NONE',  ( 0.000000000000000000, 0.000000000000000000, -1.000000000000000000 ) ) ;
#11247=EDGE_LOOP ( 'NONE', ( #6150, #3964, #15086, #8939, #7568 ) ) ;
#11249=CARTESIAN_POINT ( 'NONE',  ( 7.958171371211042455, 6.326703190994719783, -2.666481567098319960 ) ) ;
#11291=ORIENTED_EDGE ( 'NONE', *, *, #17759, .T. ) ;
#11301=CIRCLE ( 'NONE', #13643, 9.500000000000000000 ) ;
#11311=PLANE ( 'NONE',  #1470 ) ;
#11317=AXIS2_PLACEMENT_3D ( 'NONE', #946, #17576, #5096 ) ;
#11336=AXIS2_PLACEMENT_3D ( 'NONE', #143, #7409, #15278 ) ;
#11338=CIRCLE ( 'NONE', #3554, 6.000000000000000888 ) ;
#11374=ORIENTED_EDGE ( 'NONE', *, *, #11670, .T. ) ;
#11384=ORIENTED_EDGE ( 'NONE', *, *, #2220, .T. ) ;
#11406=CARTESIAN_POINT ( 'NONE',  ( 0.000000000000000000, 0.000000000000000000, -2.000000000000000000 ) ) ;
#11408=EDGE_CURVE ( 'NONE', #12324, #10066, #9551, .T. ) ;
#11421=ORIENTED_EDGE ( 'NONE', *, *, #1398, .T. ) ;
#11422=ORIENTED_EDGE ( 'NONE', *, *, #4639, .F. ) ;
#11426=ORIENTED_EDGE ( 'NONE', *, *, #10870, .T. ) ;
#11441=DIRECTION ( 'NONE',  ( -0.000000000000000000, -0.000000000000000000, -1.000000000000000000 ) ) ;
#11446=VERTEX_POINT ( 'NONE', #6572 ) ;
#11479=VERTEX_POINT ( 'NONE', #8282 ) ;
#11483=VERTEX_POINT ( 'NONE', #9543 ) ;
#11486=CIRCLE ( 'NONE', #16438, 10.50000000000000000 ) ;
#11497=DIRECTION ( 'NONE',  ( -1.000000000000000000, -1.224646799147353207E-16, 0.000000000000000000 ) ) ;
#11499=DIRECTION ( 'NONE',  ( 0.8660254037844329345, -0.5000000000000099920, 0.000000000000000000 ) ) ;
#11513=TOROIDAL_SURFACE ( 'NONE', #2566, 10.40000000000000036, 0.9000000000000003553 ) ;
#11533=CARTESIAN_POINT ( 'NONE',  ( 10.47816170930907553, -0.6768509389586216951, -6.005572809000082835 ) ) ;
#11535=CARTESIAN_POINT ( 'NONE',  ( 7.666200962222337267, 6.158133996769685758, -2.333128398347827925 ) ) ;
#11552=CIRCLE ( 'NONE', #7228, 6.000000000000000888 ) ;
#11579=CARTESIAN_POINT ( 'NONE',  ( 0.000000000000000000, 0.000000000000000000, -2.000000000000000000 ) ) ;
#11583=COLOUR_RGB ( '', 0.31764706, 0.68627451, 0.89019608) ;
#11600=DIRECTION ( 'NONE',  ( -0.06446199418653550395, -0.9979201627913403261, -4.248110196704583871E-22 ) ) ;
#11618=CARTESIAN_POINT ( 'NONE',  ( 0.000000000000000000, 0.000000000000000000, -2.000000000000000000 ) ) ;
#11621=MECHANICAL_DESIGN_GEOMETRIC_PRESENTATION_REPRESENTATION('',(#6420),#13944);
#11633=ORIENTED_EDGE ( 'NONE', *, *, #710, .T. ) ;
#11634=DIRECTION ( 'NONE',  ( 1.000000000000000000, 0.000000000000000000, 0.000000000000000000 ) ) ;
#11636=CARTESIAN_POINT ( 'NONE',  ( 0.000000000000000000, 0.000000000000000000, -10.00000000000000000 ) ) ;
#11646=CARTESIAN_POINT ( 'NONE',  ( -8.250000000000060396, -6.495190528383215423, -3.000000000000000000 ) ) ;
#11655=DIRECTION ( 'NONE',  ( 1.000000000000000000, 0.000000000000000000, 0.000000000000000000 ) ) ;
#11658=ORIENTED_EDGE ( 'NONE', *, *, #6802, .F. ) ;
#11670=EDGE_CURVE ( 'NONE', #43, #1615, #7566, .T. ) ;
#11676=CARTESIAN_POINT ( 'NONE',  ( 10.27627944162883544, 4.200961894323318013, -2.000000000000000000 ) ) ;
#11683=DIRECTION ( 'NONE',  ( 0.000000000000000000, 0.000000000000000000, -1.000000000000000000 ) ) ;
#11720=CARTESIAN_POINT ( 'NONE',  ( -10.47816170930907553, 0.6768509389586230274, -7.794427190999915211 ) ) ;
#11726=CARTESIAN_POINT ( 'NONE',  ( -2.500000000000000000, 3.061616997868383141E-16, -10.00000000000000000 ) ) ;
#11731=DIRECTION ( 'NONE',  ( -0.9979201627913402151, 0.06446199418653550395, 5.311609029246448998E-22 ) ) ;
#11734=ORIENTED_EDGE ( 'NONE', *, *, #8075, .F. ) ;
#11763=DIRECTION ( 'NONE',  ( 0.000000000000000000, 0.000000000000000000, -1.000000000000000000 ) ) ;
#11778=ORIENTED_EDGE ( 'NONE', *, *, #16958, .F. ) ;
#11823=FACE_OUTER_BOUND ( 'NONE', #11247, .T. ) ;
#11825=ORIENTED_EDGE ( 'NONE', *, *, #1512, .T. ) ;
#11830=CARTESIAN_POINT ( 'NONE',  ( -8.776279441628885181, -6.799038105676576293, -11.72793873352920890 ) ) ;
#11845=DIRECTION ( 'NONE',  ( 1.000000000000000000, 0.000000000000000000, 0.000000000000000000 ) ) ;
#11852=VECTOR ( 'NONE', #17234, 1000.000000000000000 ) ;
#11863=CIRCLE ( 'NONE', #4047, 10.50000000000000000 ) ;
#11866=DIRECTION ( 'NONE',  ( -0.9979201627913402151, 0.06446199418653550395, 5.311609029246448998E-22 ) ) ;
#11882=DIRECTION ( 'NONE',  ( 1.000000000000000000, 0.000000000000000000, 0.000000000000000000 ) ) ;
#11885=DIRECTION ( 'NONE',  ( -1.000000000000000000, -1.065814103640150279E-14, 0.000000000000000000 ) ) ;
#11889=DIRECTION ( 'NONE',  ( 0.000000000000000000, 0.000000000000000000, -1.000000000000000000 ) ) ;
#11896=CIRCLE ( 'NONE', #16536, 10.50000000000000000 ) ;
#11932=AXIS2_PLACEMENT_3D ( 'NONE', #5312, #8043, #17872 ) ;
#11945=ORIENTED_EDGE ( 'NONE', *, *, #15067, .T. ) ;
#11961=DIRECTION ( 'NONE',  ( -5.026720092345836698E-22, 4.581671729415424240E-22, -1.000000000000000000 ) ) ;
#11969=EDGE_LOOP ( 'NONE', ( #10510, #14702, #1526, #2540 ) ) ;
#11983=CARTESIAN_POINT ( 'NONE',  ( 0.000000000000000000, 0.000000000000000000, -3.000000000000000000 ) ) ;
#12033=CARTESIAN_POINT ( 'NONE',  ( 0.000000000000000000, 0.000000000000000000, -3.000000000000000000 ) ) ;
#12118=VERTEX_POINT ( 'NONE', #9251 ) ;
#12119=ORIENTED_EDGE ( 'NONE', *, *, #15355, .T. ) ;
#12150=LINE ( 'NONE', #14713, #8998 ) ;
#12159=DIRECTION ( 'NONE',  ( -1.000000000000000000, 0.000000000000000000, 0.000000000000000000 ) ) ;
#12170=EDGE_CURVE ( 'NONE', #4780, #2226, #7987, .T. ) ;
#12194=EDGE_LOOP ( 'NONE', ( #7402, #9972, #11291, #5817 ) ) ;
#12210=ADVANCED_FACE ( 'NONE', ( #9507 ), #9005, .T. ) ;
#12214=TOROIDAL_SURFACE ( 'NONE', #2389, 10.40000000000000036, 0.9000000000000003553 ) ;
#12222=CARTESIAN_POINT ( 'NONE',  ( 1.296864337298335788E-21, -1.182044466681725685E-21, -6.899999999999998579 ) ) ;
#12231=CIRCLE ( 'NONE', #16013, 10.50000000000000000 ) ;
#12243=AXIS2_PLACEMENT_3D ( 'NONE', #13884, #16029, #14661 ) ;
#12255=EDGE_CURVE ( 'NONE', #10066, #6664, #4078, .T. ) ;
#12258=PLANE ( 'NONE',  #3104 ) ;
#12275=DIRECTION ( 'NONE',  ( 1.000000000000000000, 0.000000000000000000, 0.000000000000000000 ) ) ;
#12324=VERTEX_POINT ( 'NONE', #16600 ) ;
#12332=CARTESIAN_POINT ( 'NONE',  ( 0.000000000000000000, 0.000000000000000000, -2.000000000000000000 ) ) ;
#12335=ADVANCED_FACE ( 'NONE', ( #1727 ), #5690, .T. ) ;
#12394=DIRECTION ( 'NONE',  ( 1.000000000000000000, 0.000000000000000000, -0.000000000000000000 ) ) ;
#12398=LINE ( 'NONE', #5497, #14467 ) ;
#12401=EDGE_CURVE ( 'NONE', #10034, #9359, #371, .T. ) ;
#12414=CARTESIAN_POINT ( 'NONE',  ( -1.500000000000000000, -11.00000000000000000, -9.708203932499369415 ) ) ;
#12434=DIRECTION ( 'NONE',  ( 0.000000000000000000, 0.000000000000000000, 1.000000000000000000 ) ) ;
#12441=UNCERTAINTY_MEASURE_WITH_UNIT (LENGTH_MEASURE( 1.000000000000000082E-05 ), #17825, 'distance_accuracy_value', 'NONE');
#12447=DIRECTION ( 'NONE',  ( 0.000000000000000000, 0.000000000000000000, -1.000000000000000000 ) ) ;
#12450=VERTEX_POINT ( 'NONE', #7436 ) ;
#12453=MECHANICAL_DESIGN_GEOMETRIC_PRESENTATION_REPRESENTATION('',(#10134),#6959);
#12460=DIRECTION ( 'NONE',  ( 0.000000000000000000, 0.000000000000000000, 1.000000000000000000 ) ) ;
#12473=CARTESIAN_POINT ( 'NONE',  ( -8.776279441628885181, -6.799038105676576293, -2.000000000000000000 ) ) ;
#12475=EDGE_CURVE ( 'NONE', #4593, #16631, #11301, .T. ) ;
#12479=DIRECTION ( 'NONE',  ( -0.4999999999999981126, 0.8660254037844397068, 0.000000000000000000 ) ) ;
#12485=CARTESIAN_POINT ( 'NONE',  ( 8.472608240843633681E-22, -7.722472891792491889E-22, -7.794427190999915211 ) ) ;
#12496=COLOUR_RGB ( '', 0.31764706, 0.68627451, 0.89019608) ;
#12507=CARTESIAN_POINT ( 'NONE',  ( 9.749999999999982236, -3.897114317030018871, -3.000000000000000000 ) ) ;
#12509=DIRECTION ( 'NONE',  ( 1.000000000000000000, 1.224646799147353207E-16, 0.000000000000000000 ) ) ;
#12524=ORIENTED_EDGE ( 'NONE', *, *, #8996, .T. ) ;
#12553=PLANE ( 'NONE',  #14267 ) ;
#12556=VECTOR ( 'NONE', #3331, 1000.000000000000000 ) ;
#12570=ORIENTED_EDGE ( 'NONE', *, *, #10531, .F. ) ;
#12576=PLANE ( 'NONE',  #7207 ) ;
#12580=APPLICATION_CONTEXT ( 'automotive_design' ) ;
#12588=ORIENTED_EDGE ( 'NONE', *, *, #10556, .F. ) ;
#12591=ORIENTED_EDGE ( 'NONE', *, *, #1996, .F. ) ;
#12593=ORIENTED_EDGE ( 'NONE', *, *, #6618, .T. ) ;
#12598=SHAPE_REPRESENTATION ( 'heat isolation block', ( #3575 ), #15 ) ;
#12604=DIRECTION ( 'NONE',  ( -1.000000000000000000, 0.000000000000000000, 0.000000000000000000 ) ) ;
#12609=SURFACE_SIDE_STYLE ('',( #15061 ) ) ;
#12612=CARTESIAN_POINT ( 'NONE',  ( -1.499999999999999334, 5.809475019311126864, -2.000000000000000000 ) ) ;
#12637=DIRECTION ( 'NONE',  ( 0.000000000000000000, 0.000000000000000000, -1.000000000000000000 ) ) ;
#12651=ORIENTED_EDGE ( 'NONE', *, *, #7392, .T. ) ;
#12658=CARTESIAN_POINT ( 'NONE',  ( 8.776279441628796363, -6.799038105676699750, -11.72793873352923910 ) ) ;
#12671=DIRECTION ( 'NONE',  ( -0.000000000000000000, -0.000000000000000000, -1.000000000000000000 ) ) ;
#12677=APPLICATION_CONTEXT ( 'automotive_design' ) ;
#12684=DIRECTION ( 'NONE',  ( 0.000000000000000000, 0.000000000000000000, -1.000000000000000000 ) ) ;
#12685=CIRCLE ( 'NONE', #16178, 2.500000000000000000 ) ;
#12691=DIRECTION ( 'NONE',  ( 0.8660254037844432595, 0.4999999999999921174, 0.000000000000000000 ) ) ;
#12699=EDGE_LOOP ( 'NONE', ( #2969, #10491, #11374, #4961, #4255 ) ) ;
#12746=VECTOR ( 'NONE', #10178, 1000.000000000000000 ) ;
#12766=VERTEX_POINT ( 'NONE', #9839 ) ;
#12774=EDGE_CURVE ( 'NONE', #43, #5433, #12791, .T. ) ;
#12785=DIRECTION ( 'NONE',  ( 1.224646799147353207E-16, -1.000000000000000000, 0.000000000000000000 ) ) ;
#12791=CIRCLE ( 'NONE', #15106, 10.50000000000000000 ) ;
#12794=CARTESIAN_POINT ( 'NONE',  ( 5.781152949374531502, 1.605699403978890993, -3.000000000000000888 ) ) ;
#12815=VECTOR ( 'NONE', #3306, 1000.000000000000000 ) ;
#12818=CARTESIAN_POINT ( 'NONE',  ( -10.27627944162886209, -4.200961894323246071, -2.000000000000000000 ) ) ;
#12819=VERTEX_POINT ( 'NONE', #11720 ) ;
#12820=CARTESIAN_POINT ( 'NONE',  ( 0.000000000000000000, 0.000000000000000000, -2.000000000000000000 ) ) ;
#12826=EDGE_LOOP ( 'NONE', ( #12119, #2910, #13575, #9986 ) ) ;
#12838=DIRECTION ( 'NONE',  ( -1.000000000000000000, 2.131628207280300558E-14, 0.000000000000000000 ) ) ;
#12854=AXIS2_PLACEMENT_3D ( 'NONE', #2248, #9037, #3506 ) ;
#12862=EDGE_LOOP ( 'NONE', ( #9829, #6268 ) ) ;
#12874=CARTESIAN_POINT ( 'NONE',  ( 1.296864337298335788E-21, -1.182044466681725685E-21, -6.899999999999998579 ) ) ;
#12877=LINE ( 'NONE', #12961, #4980 ) ;
#12895=CYLINDRICAL_SURFACE ( 'NONE', #1802, 6.000000000000000888 ) ;
#12901=DIRECTION ( 'NONE',  ( -0.8660254037844363761, 0.5000000000000038858, 0.000000000000000000 ) ) ;
#12903=DIRECTION ( 'NONE',  ( -0.000000000000000000, -0.000000000000000000, -1.000000000000000000 ) ) ;
#12913=ORIENTED_EDGE ( 'NONE', *, *, #12982, .F. ) ;
#12922=EDGE_CURVE ( 'NONE', #14411, #14109, #10449, .T. ) ;
#12923=EDGE_LOOP ( 'NONE', ( #10008, #10418, #17699, #17957 ) ) ;
#12930=ADVANCED_FACE ( 'NONE', ( #849 ), #6380, .F. ) ;
#12945=EDGE_CURVE ( 'NONE', #17504, #9792, #16189, .T. ) ;
#12947=PRODUCT_DEFINITION_FORMATION_WITH_SPECIFIED_SOURCE ( 'ANY', '', #3615, .NOT_KNOWN. ) ;
#12953=DIRECTION ( 'NONE',  ( 1.000000000000000000, 0.000000000000000000, 0.000000000000000000 ) ) ;
#12961=CARTESIAN_POINT ( 'NONE',  ( 1.500000000000000000, 11.00000000000000000, -3.000000000000000000 ) ) ;
#12982=EDGE_CURVE ( 'NONE', #9800, #13928, #16276, .T. ) ;
#12986=DIRECTION ( 'NONE',  ( 0.000000000000000000, 0.000000000000000000, 1.000000000000000000 ) ) ;
#12994=DIRECTION ( 'NONE',  ( 0.000000000000000000, 0.000000000000000000, 1.000000000000000000 ) ) ;
#12999=AXIS2_PLACEMENT_3D ( 'NONE', #11166, #16737, #8482 ) ;
#13010=CARTESIAN_POINT ( 'NONE',  ( 8.776279441628840772, 6.799038105676637578, -2.000000000000000000 ) ) ;
#13011=CARTESIAN_POINT ( 'NONE',  ( 0.000000000000000000, 0.000000000000000000, -10.00000000000000000 ) ) ;
#13012=DIRECTION ( 'NONE',  ( 1.000000000000000000, 0.000000000000000000, 0.000000000000000000 ) ) ;
#13049=DIRECTION ( 'NONE',  ( 0.8660254037844397068, 0.4999999999999981126, -0.000000000000000000 ) ) ;
#13063=VECTOR ( 'NONE', #13049, 1000.000000000000000 ) ;
#13077=VECTOR ( 'NONE', #16008, 999.9999999999998863 ) ;
#13100=CARTESIAN_POINT ( 'NONE',  ( -9.750000000000035527, -3.897114317029883868, -3.000000000000002665 ) ) ;
#13106=DIRECTION ( 'NONE',  ( -0.000000000000000000, -0.000000000000000000, -1.000000000000000000 ) ) ;
#13116=CARTESIAN_POINT ( 'NONE',  ( 0.000000000000000000, 0.000000000000000000, -3.000000000000000000 ) ) ;
#13117=DIRECTION ( 'NONE',  ( 0.8660254037844432595, 0.4999999999999921174, 0.000000000000000000 ) ) ;
#13130=VERTEX_POINT ( 'NONE', #9690 ) ;
#13145=VERTEX_POINT ( 'NONE', #12612 ) ;
#13147=CARTESIAN_POINT ( 'NONE',  ( 9.749999999999982236, -3.897114317030018871, -3.000000000000000000 ) ) ;
#13149=ORIENTED_EDGE ( 'NONE', *, *, #557, .F. ) ;
#13157=ADVANCED_FACE ( 'NONE', ( #15239 ), #470, .T. ) ;
#13186=FACE_BOUND ( 'NONE', #11109, .T. ) ;
#13233=EDGE_CURVE ( 'NONE', #9792, #17313, #4625, .T. ) ;
#13277=CARTESIAN_POINT ( 'NONE',  ( 0.000000000000000000, 0.000000000000000000, -2.000000000000000000 ) ) ;
#13279=ORIENTED_EDGE ( 'NONE', *, *, #557, .T. ) ;
#13309=CIRCLE ( 'NONE', #2322, 10.50000000000000000 ) ;
#13336=ORIENTED_EDGE ( 'NONE', *, *, #11408, .T. ) ;
#13345=VECTOR ( 'NONE', #9960, 999.9999999999998863 ) ;
#13371=CARTESIAN_POINT ( 'NONE',  ( 0.000000000000000000, 0.000000000000000000, -10.00000000000000000 ) ) ;
#13382=EDGE_CURVE ( 'NONE', #16631, #17480, #3715, .T. ) ;
#13385=CARTESIAN_POINT ( 'NONE',  ( 4.281152949374537720, 4.203775615332211224, -1.901951201008075243 ) ) ;
#13402=AXIS2_PLACEMENT_3D ( 'NONE', #4131, #9637, #6760 ) ;
#13407=ORIENTED_EDGE ( 'NONE', *, *, #15785, .F. ) ;
#13419=EDGE_CURVE ( 'NONE', #12118, #1069, #12685, .T. ) ;
#13425=( LENGTH_UNIT ( ) NAMED_UNIT ( * ) SI_UNIT ( .MILLI., .METRE. ) );
#13428=AXIS2_PLACEMENT_3D ( 'NONE', #15508, #14336, #16885 ) ;
#13432=DIRECTION ( 'NONE',  ( 0.000000000000000000, 0.000000000000000000, -1.000000000000000000 ) ) ;
#13436=DIRECTION ( 'NONE',  ( 0.000000000000000000, 0.000000000000000000, -1.000000000000000000 ) ) ;
#13454=CARTESIAN_POINT ( 'NONE',  ( 9.458171371211012257, -3.728626979641465500, -2.666481567098319072 ) ) ;
#13462=EDGE_LOOP ( 'NONE', ( #10837, #8899, #8244, #5379 ) ) ;
#13506=PLANE ( 'NONE',  #13965 ) ;
#13507=DIRECTION ( 'NONE',  ( 0.000000000000000000, 0.000000000000000000, -1.000000000000000000 ) ) ;
#13538=DIRECTION ( 'NONE',  ( 0.000000000000000000, 0.000000000000000000, 1.000000000000000000 ) ) ;
#13575=ORIENTED_EDGE ( 'NONE', *, *, #3292, .T. ) ;
#13626=EDGE_CURVE ( 'NONE', #8959, #13130, #8654, .T. ) ;
#13634=LINE ( 'NONE', #1580, #219 ) ;
#13643=AXIS2_PLACEMENT_3D ( 'NONE', #12874, #6055, #4701 ) ;
#13645=AXIS2_PLACEMENT_3D ( 'NONE', #16263, #11889, #7909 ) ;
#13669=ORIENTED_EDGE ( 'NONE', *, *, #2109, .T. ) ;
#13672=DIRECTION ( 'NONE',  ( 0.000000000000000000, 0.000000000000000000, 1.000000000000000000 ) ) ;
#13676=AXIS2_PLACEMENT_3D ( 'NONE', #2868, #12479, #1258 ) ;
#13705=ORIENTED_EDGE ( 'NONE', *, *, #6720, .F. ) ;
#13711=DIRECTION ( 'NONE',  ( 0.000000000000000000, 0.000000000000000000, -1.000000000000000000 ) ) ;
#13715=ADVANCED_FACE ( 'NONE', ( #4252 ), #9753, .T. ) ;
#13722=DIRECTION ( 'NONE',  ( -0.000000000000000000, -0.000000000000000000, 1.000000000000000000 ) ) ;
#13744=B_SPLINE_CURVE_WITH_KNOTS ( 'NONE', 3,
 ( #515, #15382, #1523, #1699 ),
 .UNSPECIFIED., .F., .F.,
 ( 4, 4 ),
 ( 0.007932485430080134237, 0.009354825709699442216 ),
 .UNSPECIFIED. ) ;
#13753=ORIENTED_EDGE ( 'NONE', *, *, #2462, .F. ) ;
#13763=CARTESIAN_POINT ( 'NONE',  ( 0.000000000000000000, 0.000000000000000000, -2.000000000000000000 ) ) ;
#13788=DIRECTION ( 'NONE',  ( 1.000000000000000000, 0.000000000000000000, 0.000000000000000000 ) ) ;
#13791=FILL_AREA_STYLE_COLOUR ( '', #12496 ) ;
#13805=EDGE_CURVE ( 'NONE', #9359, #6677, #5566, .T. ) ;
#13814=ORIENTED_EDGE ( 'NONE', *, *, #4099, .T. ) ;
#13831=AXIS2_PLACEMENT_3D ( 'NONE', #4534, #8533, #5613 ) ;
#13856=CARTESIAN_POINT ( 'NONE',  ( -1.500000000000000000, -10.05532945112458876, -2.666480854966549074 ) ) ;
#13864=ADVANCED_FACE ( 'NONE', ( #15464 ), #5654, .F. ) ;
#13870=CIRCLE ( 'NONE', #6046, 9.500000000000001776 ) ;
#13884=CARTESIAN_POINT ( 'NONE',  ( 10.37836969302994028, -0.6704047395399680420, -6.899999999999998579 ) ) ;
#13908=VERTEX_POINT ( 'NONE', #15917 ) ;
#13914=PRODUCT_CONTEXT ( 'NONE', #12677, 'mechanical' ) ;
#13921=EDGE_CURVE ( 'NONE', #2438, #14580, #848, .T. ) ;
#13927=DIRECTION ( 'NONE',  ( 0.000000000000000000, 0.000000000000000000, -1.000000000000000000 ) ) ;
#13928=VERTEX_POINT ( 'NONE', #7407 ) ;
#13936=CARTESIAN_POINT ( 'NONE',  ( -10.50000000000000000, 0.000000000000000000, -3.000000000000002665 ) ) ;
#13943=ORIENTED_EDGE ( 'NONE', *, *, #16776, .F. ) ;
#13944=( GEOMETRIC_REPRESENTATION_CONTEXT ( 3 ) GLOBAL_UNCERTAINTY_ASSIGNED_CONTEXT ( ( #12441 ) ) GLOBAL_UNIT_ASSIGNED_CONTEXT ( ( #17825, #11128, #16694 ) ) REPRESENTATION_CONTEXT ( 'NONE', 'WORKASPACE' ) );
#13965=AXIS2_PLACEMENT_3D ( 'NONE', #5145, #16236, #10844 ) ;
#13969=VERTEX_POINT ( 'NONE', #7484 ) ;
#13975=ADVANCED_FACE ( 'NONE', ( #6390 ), #15643, .T. ) ;
#13979=AXIS2_PLACEMENT_3D ( 'NONE', #2250, #2343, #7861 ) ;
#13984=ORIENTED_EDGE ( 'NONE', *, *, #6976, .F. ) ;
#14006=ORIENTED_EDGE ( 'NONE', *, *, #15609, .T. ) ;
#14021=CARTESIAN_POINT ( 'NONE',  ( -4.281152949374567029, -4.203775615332181026, -1.901951201008075243 ) ) ;
#14024=VERTEX_POINT ( 'NONE', #4750 ) ;
#14054=CARTESIAN_POINT ( 'NONE',  ( 0.000000000000000000, 0.000000000000000000, -1.901951201008075243 ) ) ;
#14055=EDGE_CURVE ( 'NONE', #17008, #11483, #14987, .T. ) ;
#14056=DIRECTION ( 'NONE',  ( 1.000000000000000000, 0.000000000000000000, 0.000000000000000000 ) ) ;
#14070=VERTEX_POINT ( 'NONE', #4020 ) ;
#14091=ORIENTED_EDGE ( 'NONE', *, *, #14055, .T. ) ;
#14109=VERTEX_POINT ( 'NONE', #14904 ) ;
#14128=ADVANCED_FACE ( 'NONE', ( #17667 ), #16283, .F. ) ;
#14148=PLANE ( 'NONE',  #7208 ) ;
#14184=ORIENTED_EDGE ( 'NONE', *, *, #137, .F. ) ;
#14217=CYLINDRICAL_SURFACE ( 'NONE', #842, 6.000000000000000888 ) ;
#14223=VECTOR ( 'NONE', #15719, 1000.000000000000114 ) ;
#14227=ORIENTED_EDGE ( 'NONE', *, *, #16240, .T. ) ;
#14229=PRODUCT_DEFINITION ( 'UNKNOWN', '', #12947, #1408 ) ;
#14267=AXIS2_PLACEMENT_3D ( 'NONE', #5468, #15096, #6842 ) ;
#14271=AXIS2_PLACEMENT_3D ( 'NONE', #8261, #13711, #2558 ) ;
#14272=CYLINDRICAL_SURFACE ( 'NONE', #7459, 10.50000000000000000 ) ;
#14285=CYLINDRICAL_SURFACE ( 'NONE', #5481, 6.000000000000000888 ) ;
#14287=ORIENTED_EDGE ( 'NONE', *, *, #7834, .T. ) ;
#14316=CARTESIAN_POINT ( 'NONE',  ( 1.499999999999999778, -9.380831519646861238, -2.000000000000000000 ) ) ;
#14336=DIRECTION ( 'NONE',  ( 0.000000000000000000, 0.000000000000000000, -1.000000000000000000 ) ) ;
#14350=VERTEX_POINT ( 'NONE', #7386 ) ;
#14357=CARTESIAN_POINT ( 'NONE',  ( 0.000000000000000000, 0.000000000000000000, -2.000000000000000000 ) ) ;
#14367=FACE_OUTER_BOUND ( 'NONE', #821, .T. ) ;
#14369=DIRECTION ( 'NONE',  ( 1.224646799147353207E-16, -1.000000000000000000, 0.000000000000000000 ) ) ;
#14390=LINE ( 'NONE', #13385, #667 ) ;
#14411=VERTEX_POINT ( 'NONE', #4814 ) ;
#14415=AXIS2_PLACEMENT_3D ( 'NONE', #1768, #15904, #17195 ) ;
#14420=LINE ( 'NONE', #634, #10148 ) ;
#14425=EDGE_CURVE ( 'NONE', #14580, #2839, #749, .T. ) ;
#14436=ORIENTED_EDGE ( 'NONE', *, *, #4099, .F. ) ;
#14467=VECTOR ( 'NONE', #11020, 1000.000000000000000 ) ;
#14474=CARTESIAN_POINT ( 'NONE',  ( -7.374038404636016786, -5.989453865500021124, -2.000000000000000000 ) ) ;
#14484=FACE_OUTER_BOUND ( 'NONE', #12826, .T. ) ;
#14489=CIRCLE ( 'NONE', #6653, 9.500000000000001776 ) ;
#14502=ORIENTED_EDGE ( 'NONE', *, *, #15609, .F. ) ;
#14507=DIRECTION ( 'NONE',  ( -0.000000000000000000, -0.000000000000000000, -1.000000000000000000 ) ) ;
#14508=LINE ( 'NONE', #17248, #16456 ) ;
#14519=PRESENTATION_STYLE_ASSIGNMENT (( #2374 ) ) ;
#14530=VERTEX_POINT ( 'NONE', #17470 ) ;
#14536=ADVANCED_FACE ( 'NONE', ( #932, #6468 ), #12258, .T. ) ;
#14540=CIRCLE ( 'NONE', #9312, 10.50000000000000000 ) ;
#14546=LINE ( 'NONE', #8735, #14223 ) ;
#14549=CIRCLE ( 'NONE', #2653, 6.000000000000000888 ) ;
#14551=CARTESIAN_POINT ( 'NONE',  ( 10.50000000000000000, 1.285879139104720831E-15, -2.000000000000000000 ) ) ;
#14552=VECTOR ( 'NONE', #7503, 1000.000000000000114 ) ;
#14558=DIRECTION ( 'NONE',  ( 1.000000000000000000, 0.000000000000000000, 0.000000000000000000 ) ) ;
#14565=PLANE ( 'NONE',  #6716 ) ;
#14569=EDGE_CURVE ( 'NONE', #579, #12324, #10686, .T. ) ;
#14580=VERTEX_POINT ( 'NONE', #10866 ) ;
#14596=FACE_OUTER_BOUND ( 'NONE', #13462, .T. ) ;
#14613=DIRECTION ( 'NONE',  ( 1.000000000000000000, 0.000000000000000000, 0.000000000000000000 ) ) ;
#14619=ORIENTED_EDGE ( 'NONE', *, *, #4069, .F. ) ;
#14629=CARTESIAN_POINT ( 'NONE',  ( 10.50000000000000000, 1.285879139104720831E-15, -7.794427190999915211 ) ) ;
#14656=DIRECTION ( 'NONE',  ( 0.000000000000000000, 0.000000000000000000, 1.000000000000000000 ) ) ;
#14661=DIRECTION ( 'NONE',  ( -0.9979201627913403261, 0.06446199418653535129, 0.000000000000000000 ) ) ;
#14687=ORIENTED_EDGE ( 'NONE', *, *, #7811, .T. ) ;
#14696=CARTESIAN_POINT ( 'NONE',  ( 1.296864337298335788E-21, -1.182044466681725685E-21, -6.899999999999998579 ) ) ;
#14697=( NAMED_UNIT ( * ) SI_UNIT ( $, .STERADIAN. ) SOLID_ANGLE_UNIT ( ) );
#14698=ADVANCED_FACE ( 'NONE', ( #189 ), #4555, .T. ) ;
#14702=ORIENTED_EDGE ( 'NONE', *, *, #2806, .F. ) ;
#14713=CARTESIAN_POINT ( 'NONE',  ( -6.000000000000000888, 0.000000000000000000, -1.901951201008075243 ) ) ;
#14726=EDGE_CURVE ( 'NONE', #6664, #14530, #17914, .T. ) ;
#14764=AXIS2_PLACEMENT_3D ( 'NONE', #10094, #17397, #2053 ) ;
#14785=SURFACE_SIDE_STYLE ('',( #7626 ) ) ;
#14796=DIRECTION ( 'NONE',  ( 0.000000000000000000, 0.000000000000000000, 1.000000000000000000 ) ) ;
#14810=AXIS2_PLACEMENT_3D ( 'NONE', #73, #3309, #5585 ) ;
#14814=DIRECTION ( 'NONE',  ( -1.224646799147353207E-16, 1.000000000000000000, 0.000000000000000000 ) ) ;
#14830=ORIENTED_EDGE ( 'NONE', *, *, #10359, .F. ) ;
#14840=B_SPLINE_CURVE_WITH_KNOTS ( 'NONE', 3,
 ( #13100, #3665, #6482, #10619 ),
 .UNSPECIFIED., .F., .F.,
 ( 4, 4 ),
 ( 2.843119637679310382E-07, 0.001422633878257846627 ),
 .UNSPECIFIED. ) ;
#14867=ORIENTED_EDGE ( 'NONE', *, *, #4107, .T. ) ;
#14899=ORIENTED_EDGE ( 'NONE', *, *, #12945, .T. ) ;
#14904=CARTESIAN_POINT ( 'NONE',  ( -8.250000000000060396, -6.495190528383215423, -3.000000000000000000 ) ) ;
#14927=DIRECTION ( 'NONE',  ( 1.224646799147353207E-16, -1.000000000000000000, 0.000000000000000000 ) ) ;
#14987=LINE ( 'NONE', #16452, #15615 ) ;
#15003=CYLINDRICAL_SURFACE ( 'NONE', #13402, 6.000000000000000888 ) ;
#15018=VECTOR ( 'NONE', #14369, 1000.000000000000000 ) ;
#15040=VERTEX_POINT ( 'NONE', #3957 ) ;
#15049=AXIS2_PLACEMENT_3D ( 'NONE', #15479, #3062, #8582 ) ;
#15051=DIRECTION ( 'NONE',  ( 0.8660254037844363761, -0.5000000000000038858, 0.000000000000000000 ) ) ;
#15061=SURFACE_STYLE_FILL_AREA ( #6896 ) ;
#15067=EDGE_CURVE ( 'NONE', #5433, #4593, #7015, .T. ) ;
#15072=VERTEX_POINT ( 'NONE', #3785 ) ;
#15086=ORIENTED_EDGE ( 'NONE', *, *, #15067, .F. ) ;
#15096=DIRECTION ( 'NONE',  ( -0.5000000000000099920, -0.8660254037844329345, 0.000000000000000000 ) ) ;
#15106=AXIS2_PLACEMENT_3D ( 'NONE', #12485, #15293, #71 ) ;
#15109=EDGE_LOOP ( 'NONE', ( #6455, #1938, #15306, #16730 ) ) ;
#15127=CARTESIAN_POINT ( 'NONE',  ( -10.27627944162877505, 4.200961894323461010, -2.000000000000000000 ) ) ;
#15134=ORIENTED_EDGE ( 'NONE', *, *, #13805, .F. ) ;
#15139=ORIENTED_EDGE ( 'NONE', *, *, #12170, .T. ) ;
#15178=ORIENTED_EDGE ( 'NONE', *, *, #480, .F. ) ;
#15185=DIRECTION ( 'NONE',  ( 0.000000000000000000, 0.000000000000000000, -1.000000000000000000 ) ) ;
#15189=EDGE_CURVE ( 'NONE', #1069, #12118, #1235, .T. ) ;
#15204=DIRECTION ( 'NONE',  ( 0.000000000000000000, 0.000000000000000000, -1.000000000000000000 ) ) ;
#15213=CARTESIAN_POINT ( 'NONE',  ( 8.874038404635943067, -3.391377654146811693, -2.000000000000000000 ) ) ;
#15224=ORIENTED_EDGE ( 'NONE', *, *, #6072, .T. ) ;
#15239=FACE_OUTER_BOUND ( 'NONE', #207, .T. ) ;
#15245=CARTESIAN_POINT ( 'NONE',  ( -1.500000000000000000, 10.39230484541326227, -3.000000000000000000 ) ) ;
#15259=EDGE_CURVE ( 'NONE', #17725, #12450, #12231, .T. ) ;
#15267=EDGE_LOOP ( 'NONE', ( #3697, #11658, #14867, #8417 ) ) ;
#15269=DIRECTION ( 'NONE',  ( 1.000000000000000000, 0.000000000000000000, -0.000000000000000000 ) ) ;
#15278=DIRECTION ( 'NONE',  ( 1.000000000000000000, 0.000000000000000000, 0.000000000000000000 ) ) ;
#15281=DIRECTION ( 'NONE',  ( 0.8660254037844432595, 0.4999999999999921174, 0.000000000000000000 ) ) ;
#15293=DIRECTION ( 'NONE',  ( -5.026720092345836698E-22, 4.581671729415424240E-22, -1.000000000000000000 ) ) ;
#15306=ORIENTED_EDGE ( 'NONE', *, *, #7943, .F. ) ;
#15322=EDGE_CURVE ( 'NONE', #9826, #6903, #6441, .T. ) ;
#15355=EDGE_CURVE ( 'NONE', #14109, #10285, #4904, .T. ) ;
#15357=CARTESIAN_POINT ( 'NONE',  ( 1.500000000000000000, -11.00000000000000000, -2.000000000000000000 ) ) ;
#15361=ORIENTED_EDGE ( 'NONE', *, *, #2231, .T. ) ;
#15382=CARTESIAN_POINT ( 'NONE',  ( 1.500000000000000000, -10.05532945112458876, -2.666480854966549074 ) ) ;
#15410=CARTESIAN_POINT ( 'NONE',  ( 0.000000000000000000, 0.000000000000000000, -3.000000000000000000 ) ) ;
#15429=AXIS2_PLACEMENT_3D ( 'NONE', #17599, #16298, #4946 ) ;
#15436=CONICAL_SURFACE ( 'NONE', #17791, 9.500000000000001776, 0.7853981633974465026 ) ;
#15452=VERTEX_POINT ( 'NONE', #17114 ) ;
#15462=EDGE_CURVE ( 'NONE', #5433, #14350, #6736, .T. ) ;
#15464=FACE_OUTER_BOUND ( 'NONE', #2116, .T. ) ;
#15470=EDGE_LOOP ( 'NONE', ( #3819, #4468, #17330, #15139 ) ) ;
#15475=DIRECTION ( 'NONE',  ( -1.000000000000000000, 0.000000000000000000, 0.000000000000000000 ) ) ;
#15479=CARTESIAN_POINT ( 'NONE',  ( 0.000000000000000000, 0.000000000000000000, -2.000000000000000000 ) ) ;
#15484=ORIENTED_EDGE ( 'NONE', *, *, #15462, .T. ) ;
#15490=ADVANCED_FACE ( 'NONE', ( #6689 ), #9066, .F. ) ;
#15498=ORIENTED_EDGE ( 'NONE', *, *, #15259, .T. ) ;
#15508=CARTESIAN_POINT ( 'NONE',  ( 0.000000000000000000, 0.000000000000000000, -3.000000000000002665 ) ) ;
#15510=PLANE ( 'NONE',  #15952 ) ;
#15555=ORIENTED_EDGE ( 'NONE', *, *, #12401, .F. ) ;
#15557=ORIENTED_EDGE ( 'NONE', *, *, #9354, .T. ) ;
#15595=EDGE_CURVE ( 'NONE', #7960, #4832, #6035, .T. ) ;
#15599=CARTESIAN_POINT ( 'NONE',  ( -10.27627944162886209, -4.200961894323246071, -11.72793873352920890 ) ) ;
#15609=EDGE_CURVE ( 'NONE', #5285, #1869, #15843, .T. ) ;
#15610=ORIENTED_EDGE ( 'NONE', *, *, #2645, .F. ) ;
#15615=VECTOR ( 'NONE', #1307, 1000.000000000000000 ) ;
#15624=FACE_OUTER_BOUND ( 'NONE', #6919, .T. ) ;
#15628=AXIS2_PLACEMENT_3D ( 'NONE', #13371, #13722, #12275 ) ;
#15636=CARTESIAN_POINT ( 'NONE',  ( -1.499999999999999334, 5.809475019311126864, -1.901951201008075243 ) ) ;
#15643=CYLINDRICAL_SURFACE ( 'NONE', #9246, 10.50000000000000000 ) ;
#15663=AXIS2_PLACEMENT_3D ( 'NONE', #11136, #3101, #9696 ) ;
#15667=DIRECTION ( 'NONE',  ( -1.000000000000000000, 0.000000000000000000, 0.000000000000000000 ) ) ;
#15719=DIRECTION ( 'NONE',  ( -0.8660254037844329345, 0.5000000000000099920, 0.000000000000000000 ) ) ;
#15763=FACE_OUTER_BOUND ( 'NONE', #15109, .T. ) ;
#15785=EDGE_CURVE ( 'NONE', #7830, #17725, #16583, .T. ) ;
#15787=EDGE_LOOP ( 'NONE', ( #912, #9846, #1566, #9991 ) ) ;
#15788=CARTESIAN_POINT ( 'NONE',  ( -10.37836969302994028, 0.6704047395399693743, -6.899999999999998579 ) ) ;
#15815=ORIENTED_EDGE ( 'NONE', *, *, #6425, .F. ) ;
#15826=ADVANCED_FACE ( 'NONE', ( #16038 ), #3609, .F. ) ;
#15843=LINE ( 'NONE', #16855, #9579 ) ;
#15848=ADVANCED_FACE ( 'NONE', ( #10989 ), #12553, .F. ) ;
#15871=LINE ( 'NONE', #17541, #940 ) ;
#15879=EDGE_CURVE ( 'NONE', #12766, #1421, #10814, .T. ) ;
#15896=DIRECTION ( 'NONE',  ( 0.8660254037844328234, -0.5000000000000099920, 0.000000000000000000 ) ) ;
#15899=ADVANCED_FACE ( 'NONE', ( #16643 ), #9718, .T. ) ;
#15904=DIRECTION ( 'NONE',  ( -0.000000000000000000, -0.000000000000000000, -1.000000000000000000 ) ) ;
#15917=CARTESIAN_POINT ( 'NONE',  ( 1.500000000000000000, 10.39230484541326227, -3.000000000000000000 ) ) ;
#15922=AXIS2_PLACEMENT_3D ( 'NONE', #17862, #16468, #14927 ) ;
#15925=ADVANCED_FACE ( 'NONE', ( #9464 ), #15003, .F. ) ;
#15952=AXIS2_PLACEMENT_3D ( 'NONE', #7268, #11497, #12785 ) ;
#16001=CONICAL_SURFACE ( 'NONE', #2669, 9.500000000000001776, 0.7853981633974465026 ) ;
#16008=DIRECTION ( 'NONE',  ( -0.8660254037844432595, -0.4999999999999921174, 0.000000000000000000 ) ) ;
#16013=AXIS2_PLACEMENT_3D ( 'NONE', #8569, #16933, #12838 ) ;
#16029=DIRECTION ( 'NONE',  ( 0.06446199418653537905, 0.9979201627913403261, 4.248110196704583871E-22 ) ) ;
#16034=ORIENTED_EDGE ( 'NONE', *, *, #1700, .T. ) ;
#16038=FACE_OUTER_BOUND ( 'NONE', #15470, .T. ) ;
#16052=ORIENTED_EDGE ( 'NONE', *, *, #5310, .F. ) ;
#16083=CARTESIAN_POINT ( 'NONE',  ( 1.296864337298335788E-21, -1.182044466681725685E-21, -6.899999999999998579 ) ) ;
#16088=DIRECTION ( 'NONE',  ( 0.000000000000000000, 0.000000000000000000, -1.000000000000000000 ) ) ;
#16136=EDGE_LOOP ( 'NONE', ( #16959, #417, #1867, #13753 ) ) ;
#16175=DIRECTION ( 'NONE',  ( -0.000000000000000000, -0.000000000000000000, 1.000000000000000000 ) ) ;
#16178=AXIS2_PLACEMENT_3D ( 'NONE', #8895, #1929, #6170 ) ;
#16179=EDGE_CURVE ( 'NONE', #4780, #17008, #80, .T. ) ;
#16189=LINE ( 'NONE', #3752, #5247 ) ;
#16208=EDGE_LOOP ( 'NONE', ( #152, #17216, #12651, #10414 ) ) ;
#16220=CARTESIAN_POINT ( 'NONE',  ( 8.472608240843633681E-22, -7.722472891792491889E-22, -7.794427190999915211 ) ) ;
#16230=DIRECTION ( 'NONE',  ( 1.000000000000000000, 0.000000000000000000, 0.000000000000000000 ) ) ;
#16236=DIRECTION ( 'NONE',  ( 0.000000000000000000, 0.000000000000000000, 1.000000000000000000 ) ) ;
#16240=EDGE_CURVE ( 'NONE', #6677, #3366, #14840, .T. ) ;
#16245=ORIENTED_EDGE ( 'NONE', *, *, #3357, .F. ) ;
#16261=ORIENTED_EDGE ( 'NONE', *, *, #17763, .F. ) ;
#16263=CARTESIAN_POINT ( 'NONE',  ( 0.000000000000000000, 0.000000000000000000, -3.000000000000002665 ) ) ;
#16268=VECTOR ( 'NONE', #16777, 1000.000000000000000 ) ;
#16276=LINE ( 'NONE', #13010, #5823 ) ;
#16283=CYLINDRICAL_SURFACE ( 'NONE', #15628, 2.500000000000000000 ) ;
#16298=DIRECTION ( 'NONE',  ( 5.026720092345836698E-22, -4.581671729415424240E-22, 1.000000000000000000 ) ) ;
#16319=AXIS2_PLACEMENT_3D ( 'NONE', #11175, #13927, #15475 ) ;
#16320=FACE_OUTER_BOUND ( 'NONE', #10656, .T. ) ;
#16344=ORIENTED_EDGE ( 'NONE', *, *, #4147, .T. ) ;
#16349=CARTESIAN_POINT ( 'NONE',  ( 0.000000000000000000, 0.000000000000000000, -2.000000000000000000 ) ) ;
#16354=EDGE_CURVE ( 'NONE', #2438, #13145, #3395, .T. ) ;
#16358=DIRECTION ( 'NONE',  ( 0.000000000000000000, 0.000000000000000000, 1.000000000000000000 ) ) ;
#16383=ORIENTED_EDGE ( 'NONE', *, *, #12255, .F. ) ;
#16426=CARTESIAN_POINT ( 'NONE',  ( 10.27627944162880702, -4.200961894323389956, -3.000000000000000888 ) ) ;
#16438=AXIS2_PLACEMENT_3D ( 'NONE', #9892, #17923, #7113 ) ;
#16452=CARTESIAN_POINT ( 'NONE',  ( 10.27627944162883544, 4.200961894323318013, -3.000000000000000888 ) ) ;
#16456=VECTOR ( 'NONE', #2184, 1000.000000000000000 ) ;
#16461=ORIENTED_EDGE ( 'NONE', *, *, #6720, .T. ) ;
#16468=DIRECTION ( 'NONE',  ( -1.000000000000000000, -1.224646799147353207E-16, 0.000000000000000000 ) ) ;
#16490=CARTESIAN_POINT ( 'NONE',  ( -1.499999999999999778, 9.380831519646861238, -2.000000000000000000 ) ) ;
#16536=AXIS2_PLACEMENT_3D ( 'NONE', #10590, #13432, #5155 ) ;
#16583=CIRCLE ( 'NONE', #15429, 10.50000000000000000 ) ;
#16592=CIRCLE ( 'NONE', #9334, 6.000000000000000888 ) ;
#16600=CARTESIAN_POINT ( 'NONE',  ( 1.499999999999999334, -5.809475019311126864, -3.000000000000000000 ) ) ;
#16617=DIRECTION ( 'NONE',  ( 1.000000000000000000, 0.000000000000000000, 0.000000000000000000 ) ) ;
#16631=VERTEX_POINT ( 'NONE', #2921 ) ;
#16643=FACE_OUTER_BOUND ( 'NONE', #16208, .T. ) ;
#16694=( NAMED_UNIT ( * ) SI_UNIT ( $, .STERADIAN. ) SOLID_ANGLE_UNIT ( ) );
#16707=ORIENTED_EDGE ( 'NONE', *, *, #10821, .F. ) ;
#16723=AXIS2_PLACEMENT_3D ( 'NONE', #4557, #7471, #14558 ) ;
#16730=ORIENTED_EDGE ( 'NONE', *, *, #9109, .F. ) ;
#16737=DIRECTION ( 'NONE',  ( 0.000000000000000000, 0.000000000000000000, -1.000000000000000000 ) ) ;
#16752=AXIS2_PLACEMENT_3D ( 'NONE', #15410, #369, #12953 ) ;
#16772=VECTOR ( 'NONE', #9819, 999.9999999999998863 ) ;
#16776=EDGE_CURVE ( 'NONE', #16631, #4593, #1862, .T. ) ;
#16777=DIRECTION ( 'NONE',  ( 0.000000000000000000, 0.000000000000000000, -1.000000000000000000 ) ) ;
#16784=DIRECTION ( 'NONE',  ( 0.000000000000000000, 0.000000000000000000, 1.000000000000000000 ) ) ;
#16788=DIRECTION ( 'NONE',  ( -1.000000000000000000, 0.000000000000000000, 0.000000000000000000 ) ) ;
#16793=CARTESIAN_POINT ( 'NONE',  ( -1.500000000000000666, -5.809475019311125976, -1.901951201008075243 ) ) ;
#16830=AXIS2_PLACEMENT_3D ( 'NONE', #8911, #7463, #2030 ) ;
#16842=ORIENTED_EDGE ( 'NONE', *, *, #15189, .F. ) ;
#16844=ORIENTED_EDGE ( 'NONE', *, *, #8272, .T. ) ;
#16853=EDGE_CURVE ( 'NONE', #6903, #9826, #1875, .T. ) ;
#16855=CARTESIAN_POINT ( 'NONE',  ( -1.500000000000000000, 11.00000000000000000, -3.000000000000000000 ) ) ;
#16885=DIRECTION ( 'NONE',  ( 1.000000000000000000, -1.421085471520200372E-14, 0.000000000000000000 ) ) ;
#16906=CIRCLE ( 'NONE', #9080, 6.000000000000000888 ) ;
#16914=EDGE_CURVE ( 'NONE', #2781, #3845, #937, .T. ) ;
#16933=DIRECTION ( 'NONE',  ( 5.026720092345836698E-22, -4.581671729415424240E-22, 1.000000000000000000 ) ) ;
#16938=ORIENTED_EDGE ( 'NONE', *, *, #6802, .T. ) ;
#16948=DIRECTION ( 'NONE',  ( -1.224646799147353207E-16, 1.000000000000000000, 0.000000000000000000 ) ) ;
#16958=EDGE_CURVE ( 'NONE', #4593, #17725, #6722, .T. ) ;
#16959=ORIENTED_EDGE ( 'NONE', *, *, #3292, .F. ) ;
#16988=EDGE_LOOP ( 'NONE', ( #8045, #5750, #10246, #11734 ) ) ;
#17007=DIRECTION ( 'NONE',  ( 1.000000000000000000, 4.440892098500626162E-15, 0.000000000000000000 ) ) ;
#17008=VERTEX_POINT ( 'NONE', #12794 ) ;
#17013=CARTESIAN_POINT ( 'NONE',  ( 0.000000000000000000, 0.000000000000000000, -3.000000000000000000 ) ) ;
#17028=ORIENTED_EDGE ( 'NONE', *, *, #17446, .F. ) ;
#17040=DIRECTION ( 'NONE',  ( 0.000000000000000000, 0.000000000000000000, -1.000000000000000000 ) ) ;
#17098=FACE_OUTER_BOUND ( 'NONE', #9612, .T. ) ;
#17102=LINE ( 'NONE', #4655, #3848 ) ;
#17112=DIRECTION ( 'NONE',  ( -1.000000000000000000, 0.000000000000000000, 0.000000000000000000 ) ) ;
#17114=CARTESIAN_POINT ( 'NONE',  ( -9.749999999999953815, 3.897114317030088149, -3.000000000000000000 ) ) ;
#17119=EDGE_LOOP ( 'NONE', ( #5922, #14091, #12588, #15178, #5134, #13669, #8265, #14502, #17633, #10816, #10119, #3405, #13279, #9755, #5329, #8857, #1332, #6462, #509, #17579, #3525, #13336, #17789, #16261, #17454 ) ) ;
#17145=ORIENTED_EDGE ( 'NONE', *, *, #6425, .T. ) ;
#17147=ORIENTED_EDGE ( 'NONE', *, *, #13382, .T. ) ;
#17179=DIRECTION ( 'NONE',  ( 0.000000000000000000, 0.000000000000000000, -1.000000000000000000 ) ) ;
#17195=DIRECTION ( 'NONE',  ( -1.000000000000000000, 0.000000000000000000, 0.000000000000000000 ) ) ;
#17208=CARTESIAN_POINT ( 'NONE',  ( -1.500000000000000666, -5.809475019311125976, -2.000000000000000000 ) ) ;
#17211=B_SPLINE_CURVE_WITH_KNOTS ( 'NONE', 3,
 ( #1360, #5333, #17894, #2637 ),
 .UNSPECIFIED., .F., .F.,
 ( 4, 4 ),
 ( 2.843119637683901301E-07, 0.001422633878257846193 ),
 .UNSPECIFIED. ) ;
#17216=ORIENTED_EDGE ( 'NONE', *, *, #14425, .T. ) ;
#17234=DIRECTION ( 'NONE',  ( -0.000000000000000000, -0.000000000000000000, -1.000000000000000000 ) ) ;
#17248=CARTESIAN_POINT ( 'NONE',  ( -10.50000000000000000, 0.000000000000000000, -2.000000000000000000 ) ) ;
#17278=CARTESIAN_POINT ( 'NONE',  ( -8.776279441628744848, 6.799038105676760146, -2.000000000000000000 ) ) ;
#17282=EDGE_CURVE ( 'NONE', #13969, #8628, #16906, .T. ) ;
#17307=ORIENTED_EDGE ( 'NONE', *, *, #16354, .T. ) ;
#17313=VERTEX_POINT ( 'NONE', #8494 ) ;
#17330=ORIENTED_EDGE ( 'NONE', *, *, #578, .T. ) ;
#17353=CIRCLE ( 'NONE', #16752, 6.000000000000000888 ) ;
#17358=EDGE_CURVE ( 'NONE', #11446, #11147, #10239, .T. ) ;
#17379=VECTOR ( 'NONE', #130, 1000.000000000000114 ) ;
#17387=PRODUCT_DEFINITION_SHAPE ( 'NONE', 'NONE',  #14229 ) ;
#17397=DIRECTION ( 'NONE',  ( 0.000000000000000000, 0.000000000000000000, 1.000000000000000000 ) ) ;
#17400=DIRECTION ( 'NONE',  ( 1.000000000000000000, 0.000000000000000000, 0.000000000000000000 ) ) ;
#17401=CARTESIAN_POINT ( 'NONE',  ( 1.296864337298335788E-21, -1.182044466681725685E-21, -6.899999999999998579 ) ) ;
#17435=CARTESIAN_POINT ( 'NONE',  ( -1.499999999999999112, 5.809475019311125976, -3.000000000000000000 ) ) ;
#17446=EDGE_CURVE ( 'NONE', #6903, #12118, #2071, .T. ) ;
#17454=ORIENTED_EDGE ( 'NONE', *, *, #12170, .F. ) ;
#17463=CIRCLE ( 'NONE', #3830, 10.50000000000000000 ) ;
#17470=CARTESIAN_POINT ( 'NONE',  ( 7.374038404635931521, -5.989453865500120600, -2.000000000000000000 ) ) ;
#17476=EDGE_LOOP ( 'NONE', ( #6554, #6223, #1993, #12570 ) ) ;
#17480=VERTEX_POINT ( 'NONE', #8020 ) ;
#17500=DIRECTION ( 'NONE',  ( -5.026720092345836698E-22, 4.581671729415424240E-22, -1.000000000000000000 ) ) ;
#17504=VERTEX_POINT ( 'NONE', #10558 ) ;
#17532=ORIENTED_EDGE ( 'NONE', *, *, #5330, .T. ) ;
#17541=CARTESIAN_POINT ( 'NONE',  ( 1.500000000000000000, 11.00000000000000000, -2.000000000000000000 ) ) ;
#17566=DIRECTION ( 'NONE',  ( 1.000000000000000000, 0.000000000000000000, -0.000000000000000000 ) ) ;
#17575=DIRECTION ( 'NONE',  ( 0.000000000000000000, 0.000000000000000000, 1.000000000000000000 ) ) ;
#17576=DIRECTION ( 'NONE',  ( 1.000000000000000000, 1.224646799147353207E-16, 0.000000000000000000 ) ) ;
#17579=ORIENTED_EDGE ( 'NONE', *, *, #17358, .F. ) ;
#17595=ORIENTED_EDGE ( 'NONE', *, *, #4191, .T. ) ;
#17599=CARTESIAN_POINT ( 'NONE',  ( 1.746467850512308208E-21, -1.591841644184202181E-21, -6.005572809000082835 ) ) ;
#17609=DIRECTION ( 'NONE',  ( 0.000000000000000000, 0.000000000000000000, -1.000000000000000000 ) ) ;
#17633=ORIENTED_EDGE ( 'NONE', *, *, #5099, .T. ) ;
#17635=CARTESIAN_POINT ( 'NONE',  ( -8.249999999999923617, 6.495190528383386841, -3.000000000000002665 ) ) ;
#17641=DIRECTION ( 'NONE',  ( 0.8660254037844363761, -0.5000000000000038858, 0.000000000000000000 ) ) ;
#17667=FACE_OUTER_BOUND ( 'NONE', #2196, .T. ) ;
#17670=CIRCLE ( 'NONE', #10932, 9.500000000000001776 ) ;
#17699=ORIENTED_EDGE ( 'NONE', *, *, #13921, .F. ) ;
#17725=VERTEX_POINT ( 'NONE', #11533 ) ;
#17738=DIRECTION ( 'NONE',  ( 1.000000000000000000, 5.329070518200751394E-15, 0.000000000000000000 ) ) ;
#17759=EDGE_CURVE ( 'NONE', #7588, #3845, #674, .T. ) ;
#17763=EDGE_CURVE ( 'NONE', #2226, #6664, #2125, .T. ) ;
#17770=ORIENTED_EDGE ( 'NONE', *, *, #3769, .T. ) ;
#17789=ORIENTED_EDGE ( 'NONE', *, *, #12255, .T. ) ;
#17791=AXIS2_PLACEMENT_3D ( 'NONE', #1984, #1626, #15667 ) ;
#17825=( LENGTH_UNIT ( ) NAMED_UNIT ( * ) SI_UNIT ( .MILLI., .METRE. ) );
#17826=CARTESIAN_POINT ( 'NONE',  ( 1.499999999999999334, -5.809475019311126864, -1.901951201008075243 ) ) ;
#17843=EDGE_CURVE ( 'NONE', #12324, #11446, #17102, .T. ) ;
#17857=EDGE_CURVE ( 'NONE', #7588, #13928, #16592, .T. ) ;
#17862=CARTESIAN_POINT ( 'NONE',  ( 1.500000000000000000, 11.00000000000000000, -9.708203932499369415 ) ) ;
#17872=DIRECTION ( 'NONE',  ( 1.000000000000000000, 0.000000000000000000, 0.000000000000000000 ) ) ;
#17880=PLANE ( 'NONE',  #7283 ) ;
#17890=CARTESIAN_POINT ( 'NONE',  ( -1.500000000000000000, -10.39230484541326405, -3.000000000000002665 ) ) ;
#17894=CARTESIAN_POINT ( 'NONE',  ( 9.166200962222330162, 3.560057785416366194, -2.333128398347829258 ) ) ;
#17897=DIRECTION ( 'NONE',  ( 0.000000000000000000, 0.000000000000000000, -1.000000000000000000 ) ) ;
#17911=DIRECTION ( 'NONE',  ( -5.026720092345836698E-22, 4.581671729415424240E-22, -1.000000000000000000 ) ) ;
#17914=B_SPLINE_CURVE_WITH_KNOTS ( 'NONE', 3,
 ( #104, #1372, #3008, #5438 ),
 .UNSPECIFIED., .F., .F.,
 ( 4, 4 ),
 ( 2.843119637679310382E-07, 0.001422633878257848579 ),
 .UNSPECIFIED. ) ;
#17923=DIRECTION ( 'NONE',  ( 0.000000000000000000, 0.000000000000000000, -1.000000000000000000 ) ) ;
#17946=LINE ( 'NONE', #12473, #6667 ) ;
#17957=ORIENTED_EDGE ( 'NONE', *, *, #752, .F. ) ;
ENDSEC;
END-ISO-10303-21;
